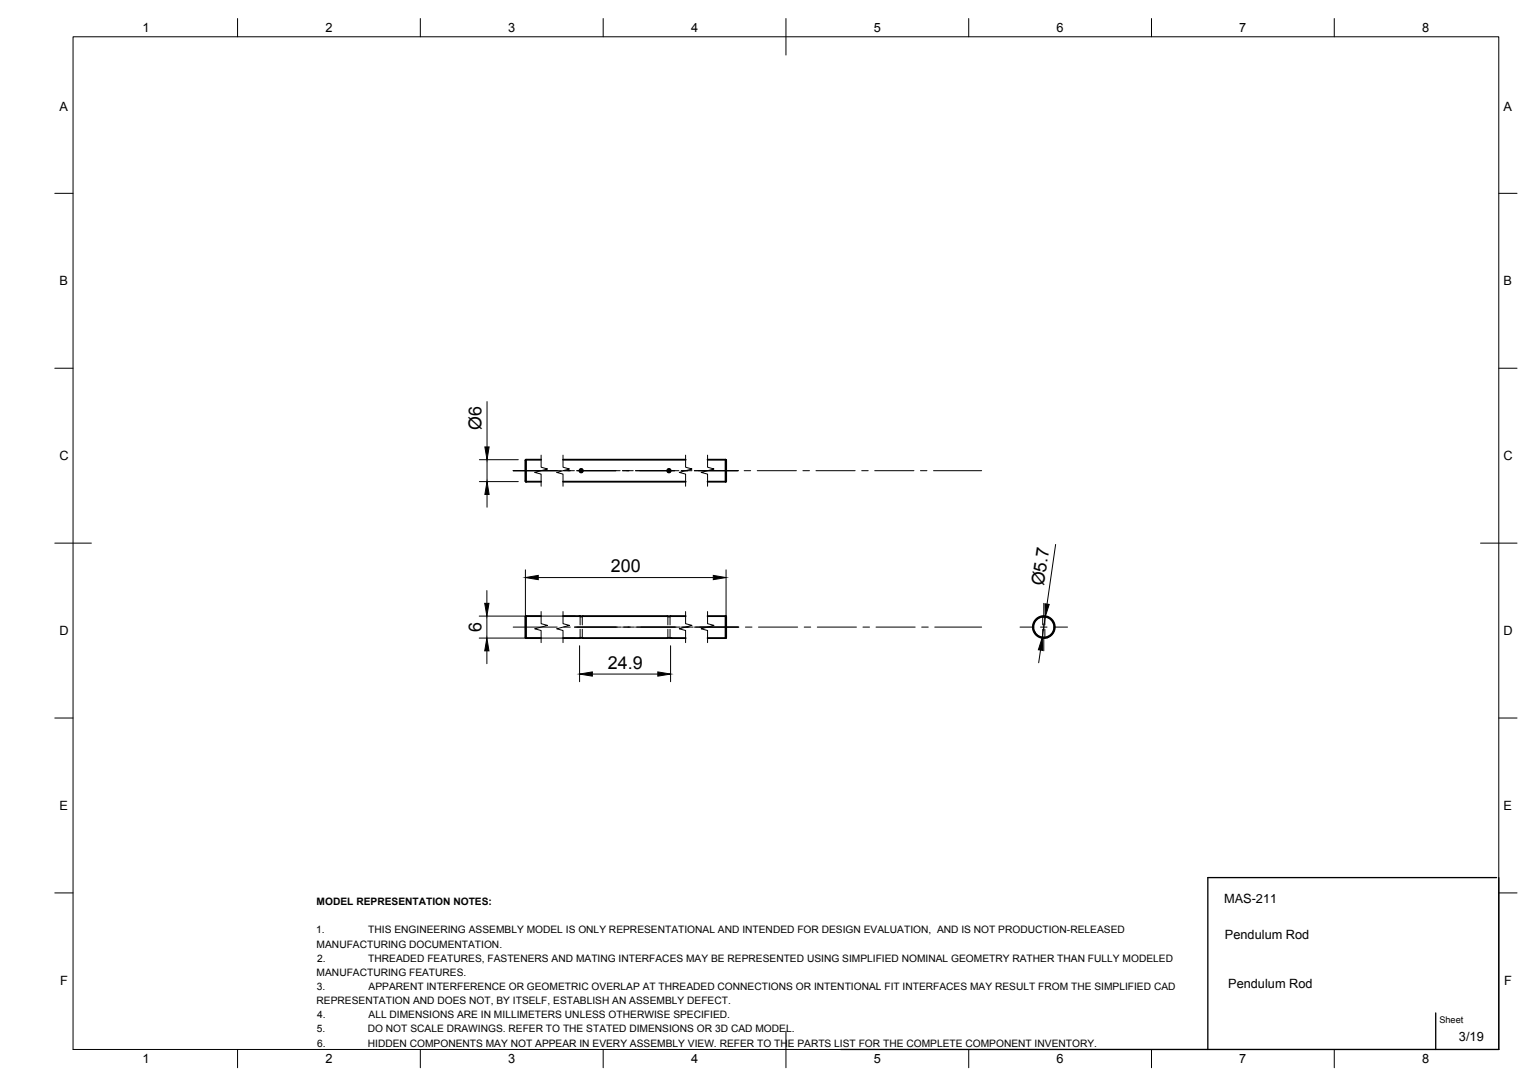
ISO-10303-21;
HEADER;
FILE_DESCRIPTION(
 (''),
 '2;1');
FILE_NAME ( 'Pendulum Rod.step', '2026-10-05T20:07:59+06:00', ( '' ), ( '' ), 'STEP AP214', 'Unspecified', '' );
FILE_SCHEMA (('AUTOMOTIVE_DESIGN { 1 0 10303 214 3 1 1 }'));
ENDSEC;
DATA;
#10=MECHANICAL_DESIGN_GEOMETRIC_PRESENTATION_REPRESENTATION('',(#319),#196741);
#319=STYLED_ITEM('',(#196765),#338) ;
#338=MANIFOLD_SOLID_BREP('Pendulum Rod',#8715) ;
#357=PLANE('',#8753) ;
#358=PLANE('',#8754) ;
#554=FACE_BOUND('',#1339,.T.) ;
#555=FACE_BOUND('',#1340,.T.) ;
#556=FACE_BOUND('',#1341,.T.) ;
#557=FACE_BOUND('',#1342,.T.) ;
#612=CIRCLE('',#8751,2.99999999999999) ;
#613=CIRCLE('',#8752,2.99999999999999) ;
#811=B_SPLINE_SURFACE_WITH_KNOTS('',1,3,((#12126,#12127,#12128,#12129,#12130,
#12131,#12132,#12133,#12134,#12135,#12136,#12137,#12138,#12139,#12140),
(#12141,#12142,#12143,#12144,#12145,#12146,#12147,#12148,#12149,#12150,
#12151,#12152,#12153,#12154,#12155)),.UNSPECIFIED.,.F.,.T.,.F.,(2,2),(4,
1,1,1,1,1,1,1,1,1,1,1,4),(-8.8354979436913E-5,0.241230871771051),(0.,0.433069184072941,
0.613631069879533,0.707969844415473,0.800502285413489,0.982878828682618,
1.41593872955056,1.84899944094778,2.03137686036412,2.12390982409441,2.21644278782049,
2.39882020722706,2.83187996119986),.UNSPECIFIED.) ;
#812=B_SPLINE_SURFACE_WITH_KNOTS('',1,3,((#12173,#12174,#12175,#12176,#12177,
#12178,#12179,#12180,#12181,#12182,#12183,#12184,#12185,#12186,#12187),
(#12188,#12189,#12190,#12191,#12192,#12193,#12194,#12195,#12196,#12197,
#12198,#12199,#12200,#12201,#12202)),.UNSPECIFIED.,.F.,.T.,.F.,(2,2),(4,
1,1,1,1,1,1,1,1,1,1,1,4),(-8.82843032138443E-5,0.241231935350036),(0.,0.433059753999551,
0.615437173415573,0.707970137120889,0.802309447772199,0.982872196325326,
1.41594123358707,1.84900113443533,2.03137767770577,2.12391011870702,2.21824889324341,
2.39881077905672,2.83187996310763),.UNSPECIFIED.) ;
#813=B_SPLINE_SURFACE_WITH_KNOTS('',1,3,((#12220,#12221,#12222,#12223,#12224,
#12225,#12226,#12227,#12228,#12229,#12230,#12231,#12232,#12233,#12234),
(#12235,#12236,#12237,#12238,#12239,#12240,#12241,#12242,#12243,#12244,
#12245,#12246,#12247,#12248,#12249)),.UNSPECIFIED.,.F.,.T.,.F.,(2,2),(4,
1,1,1,1,1,1,1,1,1,1,1,4),(-8.85365464214024E-5,0.241919354715635),(0.,0.433059753978827,
0.615437173388124,0.707970137104854,0.802309447755686,0.982872196316439,
1.41594123355621,1.84900113442618,2.03137767770062,2.12391011869139,2.21824889322736,
2.39881077903564,2.83187996310738),.UNSPECIFIED.) ;
#814=B_SPLINE_SURFACE_WITH_KNOTS('',1,3,((#12267,#12268,#12269,#12270,#12271,
#12272,#12273,#12274,#12275,#12276,#12277,#12278,#12279,#12280,#12281),
(#12282,#12283,#12284,#12285,#12286,#12287,#12288,#12289,#12290,#12291,
#12292,#12293,#12294,#12295,#12296)),.UNSPECIFIED.,.F.,.T.,.F.,(2,2),(4,
1,1,1,1,1,1,1,1,1,1,1,4),(-8.86192306118932E-5,0.241918274947197),(0.,0.433069184052406,
0.61363106986425,0.707969844400602,0.800502285411225,0.982878828678875,
1.41593872952055,1.849007766784,2.02957051533547,2.12390982598676,2.21644278969928,
2.39882020911001,2.83187996310763),.UNSPECIFIED.) ;
#815=B_SPLINE_SURFACE_WITH_KNOTS('',1,3,((#12362,#12363,#12364,#12365,#12366,
#12367,#12368,#12369,#12370,#12371,#12372,#12373,#12374,#12375,#12376,#12377,
#12378,#12379,#12380),(#12381,#12382,#12383,#12384,#12385,#12386,#12387,
#12388,#12389,#12390,#12391,#12392,#12393,#12394,#12395,#12396,#12397,#12398,
#12399)),.UNSPECIFIED.,.F.,.T.,.F.,(2,2),(4,1,1,1,1,1,1,1,1,1,1,1,1,1,1,
1,4),(0.,0.214916064382941),(0.,1.11916410687735,2.23832821375471,3.35749232063191,
4.47665642750911,5.59582053438647,6.71498464126383,7.83414874814102,8.95331285501821,
10.0724769618908,11.1916410687635,12.3108051756408,13.4299692825182,14.5491333893954,
15.6682974962725,16.7874616031499,17.9066257100273),.UNSPECIFIED.) ;
#816=B_SPLINE_SURFACE_WITH_KNOTS('',3,1,((#12401,#12402),(#12403,#12404),
(#12405,#12406),(#12407,#12408),(#12409,#12410),(#12411,#12412),(#12413,
#12414),(#12415,#12416),(#12417,#12418),(#12419,#12420),(#12421,#12422),
(#12423,#12424),(#12425,#12426),(#12427,#12428),(#12429,#12430),(#12431,
#12432),(#12433,#12434),(#12435,#12436),(#12437,#12438)),.UNSPECIFIED.,
 .T.,.F.,.F.,(4,1,1,1,1,1,1,1,1,1,1,1,1,1,1,1,4),(2,2),(0.,1.11916410687736,
2.23832821375472,3.35749232063194,4.47665642750915,5.5958205343865,6.71498464126385,
7.83414874813648,8.95331285500911,10.0724769618863,11.1916410687635,12.3108051756408,
13.4299692825181,14.5491333893953,15.6682974962725,16.7874616031499,17.9066257100273),
(0.,0.214916064382901),.UNSPECIFIED.) ;
#859=FACE_OUTER_BOUND('',#1332,.T.) ;
#860=FACE_OUTER_BOUND('',#1333,.T.) ;
#861=FACE_OUTER_BOUND('',#1334,.T.) ;
#862=FACE_OUTER_BOUND('',#1335,.T.) ;
#863=FACE_OUTER_BOUND('',#1336,.T.) ;
#864=FACE_OUTER_BOUND('',#1337,.T.) ;
#865=FACE_OUTER_BOUND('',#1338,.T.) ;
#866=FACE_OUTER_BOUND('',#1343,.T.) ;
#867=FACE_OUTER_BOUND('',#1344,.T.) ;
#868=FACE_OUTER_BOUND('',#1345,.T.) ;
#869=FACE_OUTER_BOUND('',#1346,.T.) ;
#1332=EDGE_LOOP('',(#5568,#5569,#5570,#5571,#5572,#5573)) ;
#1333=EDGE_LOOP('',(#5574,#5575,#5576,#5577,#5578,#5579)) ;
#1334=EDGE_LOOP('',(#5580,#5581,#5582,#5583,#5584)) ;
#1335=EDGE_LOOP('',(#5585,#5586,#5587,#5588,#5589)) ;
#1336=EDGE_LOOP('',(#5590,#5591,#5592,#5593,#5594)) ;
#1337=EDGE_LOOP('',(#5595,#5596,#5597,#5598,#5599)) ;
#1338=EDGE_LOOP('',(#5600,#5601,#5602,#5603)) ;
#1339=EDGE_LOOP('',(#5604)) ;
#1340=EDGE_LOOP('',(#5605)) ;
#1341=EDGE_LOOP('',(#5606)) ;
#1342=EDGE_LOOP('',(#5607)) ;
#1343=EDGE_LOOP('',(#5608)) ;
#1344=EDGE_LOOP('',(#5609)) ;
#1345=EDGE_LOOP('',(#5610,#5611,#5612,#5613)) ;
#1346=EDGE_LOOP('',(#5614,#5615,#5616,#5617)) ;
#1863=LINE('',#11652,#2566) ;
#1864=LINE('',#11926,#2567) ;
#1865=LINE('',#12157,#2568) ;
#1866=LINE('',#12204,#2569) ;
#1867=LINE('',#12251,#2570) ;
#1868=LINE('',#12298,#2571) ;
#1869=LINE('',#12318,#2572) ;
#1870=LINE('',#12400,#2573) ;
#1871=LINE('',#12439,#2574) ;
#2566=VECTOR('',#9461,0.300000000000011) ;
#2567=VECTOR('',#9464,0.299999999999991) ;
#2568=VECTOR('',#9465,10.) ;
#2569=VECTOR('',#9466,10.) ;
#2570=VECTOR('',#9467,10.) ;
#2571=VECTOR('',#9468,10.) ;
#2572=VECTOR('',#9473,3.00000000000003) ;
#2573=VECTOR('',#9480,10.) ;
#2574=VECTOR('',#9481,10.) ;
#3269=B_SPLINE_CURVE_WITH_KNOTS('',3,(#11581,#11582,#11583,#11584,#11585,
#11586,#11587,#11588,#11589,#11590,#11591,#11592,#11593,#11594,#11595,#11596,
#11597,#11598,#11599,#11600,#11601,#11602,#11603,#11604,#11605,#11606,#11607,
#11608,#11609,#11610,#11611,#11612,#11613,#11614,#11615,#11616,#11617,#11618,
#11619,#11620,#11621,#11622,#11623,#11624,#11625,#11626,#11627,#11628,#11629,
#11630,#11631,#11632,#11633,#11634,#11635,#11636,#11637,#11638,#11639,#11640,
#11641,#11642,#11643,#11644,#11645,#11646,#11647,#11648,#11649,#11650),
 .UNSPECIFIED.,.F.,.F.,(4,3,3,3,3,3,3,3,3,3,3,3,3,3,3,3,3,3,3,3,3,3,3,4),
(0.,0.0793197138435201,0.158771385884217,0.238558484111915,0.306313523372651,
0.403832448656896,0.433069184072941,0.511729267835096,0.590263878581832,
0.613631069879533,0.690390876330624,0.707969844415473,0.800502285413489,
0.876862882016797,0.95333936184816,0.982878828682618,1.06189090503122,1.14078623960736,
1.21960243454601,1.29840986633391,1.32860366242735,1.39861936931628,1.41593872955056,
1.41596897684906),.UNSPECIFIED.) ;
#3270=B_SPLINE_CURVE_WITH_KNOTS('',3,(#11654,#11655,#11656,#11657,#11658,
#11659,#11660,#11661,#11662,#11663,#11664,#11665,#11666,#11667,#11668,#11669,
#11670,#11671,#11672,#11673,#11674,#11675,#11676,#11677,#11678,#11679,#11680,
#11681,#11682,#11683,#11684,#11685,#11686,#11687,#11688,#11689,#11690,#11691,
#11692,#11693,#11694,#11695,#11696,#11697,#11698,#11699,#11700,#11701,#11702,
#11703,#11704,#11705,#11706,#11707,#11708,#11709,#11710,#11711,#11712,#11713,
#11714,#11715,#11716,#11717),.UNSPECIFIED.,.F.,.F.,(4,3,3,3,3,3,3,3,3,3,
3,3,3,3,3,3,3,3,3,3,3,4),(1.41596880340121,1.49262148871634,1.5668573581781,
1.64471845141992,1.72257954466174,1.80445466514378,1.84900113443533,1.92515260613569,
2.0012049728828,2.03137767770577,2.12391011870702,2.19942692290802,2.21824889324341,
2.29711576720828,2.37613469075668,2.39881077905672,2.48964910629467,2.58046623905025,
2.67010886019969,2.72490396964329,2.79646171749926,2.83187996310763),
 .UNSPECIFIED.) ;
#3271=B_SPLINE_CURVE_WITH_KNOTS('',3,(#11718,#11719,#11720,#11721,#11722,
#11723,#11724,#11725,#11726,#11727,#11728,#11729,#11730,#11731,#11732,#11733,
#11734,#11735,#11736,#11737,#11738,#11739,#11740,#11741,#11742,#11743,#11744,
#11745,#11746,#11747,#11748,#11749,#11750,#11751,#11752,#11753,#11754,#11755,
#11756,#11757,#11758,#11759,#11760,#11761,#11762,#11763,#11764,#11765,#11766,
#11767,#11768,#11769,#11770,#11771,#11772,#11773,#11774,#11775,#11776,#11777,
#11778,#11779,#11780,#11781,#11782,#11783,#11784,#11785,#11786,#11787),
 .UNSPECIFIED.,.F.,.F.,(4,3,3,3,3,3,3,3,3,3,3,3,3,3,3,3,3,3,3,3,3,3,3,4),
(0.,0.0793133374912053,0.158758235390486,0.238538175205765,0.306301524869595,
0.403803180865383,0.433059753999551,0.511690783685005,0.590197964800243,
0.615437173415573,0.692151852374993,0.707970137120889,0.802309447772199,
0.878720775265787,0.955248849211538,0.982872196325326,1.06188787249591,
1.14078682148802,1.21960661441308,1.2984175189742,1.32858362623266,1.39860014615873,
1.41594123358707,1.41596880340121),.UNSPECIFIED.) ;
#3272=B_SPLINE_CURVE_WITH_KNOTS('',3,(#11788,#11789,#11790,#11791,#11792,
#11793,#11794,#11795,#11796,#11797,#11798,#11799,#11800,#11801,#11802,#11803,
#11804,#11805,#11806,#11807,#11808,#11809,#11810,#11811,#11812,#11813,#11814,
#11815,#11816,#11817,#11818,#11819,#11820,#11821,#11822,#11823,#11824,#11825,
#11826,#11827,#11828,#11829,#11830,#11831,#11832,#11833,#11834,#11835,#11836,
#11837,#11838,#11839,#11840,#11841,#11842,#11843,#11844,#11845,#11846,#11847,
#11848,#11849,#11850,#11851),.UNSPECIFIED.,.F.,.F.,(4,3,3,3,3,3,3,3,3,3,
3,3,3,3,3,3,3,3,3,3,3,4),(1.41596897684906,1.49265653903016,1.56689293584109,
1.64480608070727,1.72271922557345,1.80458348138907,1.84899944094778,1.92515534328894,
2.0012121330888,2.03137686036412,2.12390982409441,2.19935680708818,2.21644278782049,
2.2952634447841,2.37423511805567,2.39882020722706,2.48964792234117,2.58045374598227,
2.6700867011423,2.72489655815223,2.79645311316558,2.83187996119986),
 .UNSPECIFIED.) ;
#3273=B_SPLINE_CURVE_WITH_KNOTS('',3,(#11855,#11856,#11857,#11858,#11859,
#11860,#11861,#11862,#11863,#11864,#11865,#11866,#11867,#11868,#11869,#11870,
#11871,#11872,#11873,#11874,#11875,#11876,#11877,#11878,#11879,#11880,#11881,
#11882,#11883,#11884,#11885,#11886,#11887,#11888,#11889,#11890,#11891,#11892,
#11893,#11894,#11895,#11896,#11897,#11898,#11899,#11900,#11901,#11902,#11903,
#11904,#11905,#11906,#11907,#11908,#11909,#11910,#11911,#11912,#11913,#11914,
#11915,#11916,#11917,#11918,#11919,#11920,#11921,#11922,#11923,#11924),
 .UNSPECIFIED.,.F.,.F.,(4,3,3,3,3,3,3,3,3,3,3,3,3,3,3,3,3,3,3,3,3,3,3,4),
(0.,0.0793133370868211,0.158758234556949,0.238538173913318,0.306301520321067,
0.403803175477182,0.433059753978827,0.511690783698259,0.590197964845532,
0.615437173388124,0.692151852363811,0.707970137104854,0.802309447755686,
0.87872077528125,0.955248849259362,0.982872196316439,1.06188787193309,1.14078682038421,
1.21960661277611,1.29841751684233,1.32858364651257,1.39860016603356,1.41594123355621,
1.41596880335427),.UNSPECIFIED.) ;
#3274=B_SPLINE_CURVE_WITH_KNOTS('',3,(#11928,#11929,#11930,#11931,#11932,
#11933,#11934,#11935,#11936,#11937,#11938,#11939,#11940,#11941,#11942,#11943,
#11944,#11945,#11946,#11947,#11948,#11949,#11950,#11951,#11952,#11953,#11954,
#11955,#11956,#11957,#11958,#11959,#11960,#11961,#11962,#11963,#11964,#11965,
#11966,#11967,#11968,#11969,#11970,#11971,#11972,#11973,#11974,#11975,#11976,
#11977,#11978,#11979,#11980,#11981,#11982,#11983,#11984,#11985,#11986,#11987,
#11988,#11989,#11990,#11991),.UNSPECIFIED.,.F.,.F.,(4,3,3,3,3,3,3,3,3,3,
3,3,3,3,3,3,3,3,3,3,3,4),(1.41596956338659,1.49266311646134,1.56690058990888,
1.64482218279723,1.72274377568557,1.80460850560754,1.849007766784,1.92524484137593,
2.00137969415775,2.02957051533547,2.12390982598676,2.19939955812894,2.21644278969928,
2.29526521978404,2.37423861455297,2.39882020911001,2.48964647817264,2.58045077014705,
2.67008242771561,2.72489376468843,2.79645019556297,2.83187996310763),
 .UNSPECIFIED.) ;
#3275=B_SPLINE_CURVE_WITH_KNOTS('',3,(#11992,#11993,#11994,#11995,#11996,
#11997,#11998,#11999,#12000,#12001,#12002,#12003,#12004,#12005,#12006,#12007,
#12008,#12009,#12010,#12011,#12012,#12013,#12014,#12015,#12016,#12017,#12018,
#12019,#12020,#12021,#12022,#12023,#12024,#12025,#12026,#12027,#12028,#12029,
#12030,#12031,#12032,#12033,#12034,#12035,#12036,#12037,#12038,#12039,#12040,
#12041,#12042,#12043,#12044,#12045,#12046,#12047,#12048,#12049,#12050,#12051,
#12052,#12053,#12054,#12055,#12056,#12057,#12058,#12059,#12060,#12061),
 .UNSPECIFIED.,.F.,.F.,(4,3,3,3,3,3,3,3,3,3,3,3,3,3,3,3,3,3,3,3,3,3,3,4),
(0.,0.0793198911693566,0.158771759312593,0.238559074159999,0.306312735619829,
0.403832566518769,0.433069184052406,0.511730463050406,0.590266238023745,
0.61363106986425,0.690383033927815,0.707969844400602,0.800502285411225,
0.876854197724648,0.953321820846053,0.982878828678875,1.06189673932164,
1.14079797822371,1.21962007756801,1.29843326555185,1.32859538269108,1.3986125617673,
1.41593872952055,1.41596956338659),.UNSPECIFIED.) ;
#3276=B_SPLINE_CURVE_WITH_KNOTS('',3,(#12062,#12063,#12064,#12065,#12066,
#12067,#12068,#12069,#12070,#12071,#12072,#12073,#12074,#12075,#12076,#12077,
#12078,#12079,#12080,#12081,#12082,#12083,#12084,#12085,#12086,#12087,#12088,
#12089,#12090,#12091,#12092,#12093,#12094,#12095,#12096,#12097,#12098,#12099,
#12100,#12101,#12102,#12103,#12104,#12105,#12106,#12107,#12108,#12109,#12110,
#12111,#12112,#12113,#12114,#12115,#12116,#12117,#12118,#12119,#12120,#12121,
#12122,#12123,#12124,#12125),.UNSPECIFIED.,.F.,.F.,(4,3,3,3,3,3,3,3,3,3,
3,3,3,3,3,3,3,3,3,3,3,4),(1.41596880335427,1.49262163677989,1.56685751827755,
1.64471882766714,1.72258013705673,1.80445525976957,1.84900113442618,1.92515260611125,
2.00120497284308,2.03137767770062,2.12391011869139,2.19942692303724,2.21824889322736,
2.29711576705383,2.37613469046074,2.39881077903564,2.48964909647063,2.58046621914314,
2.67010883124273,2.72490414691485,2.79646188868388,2.83187996310738),
 .UNSPECIFIED.) ;
#3277=B_SPLINE_CURVE_WITH_KNOTS('',3,(#12158,#12159,#12160,#12161,#12162,
#12163,#12164,#12165,#12166,#12167,#12168,#12169,#12170,#12171,#12172),
 .UNSPECIFIED.,.T.,.F.,(4,1,1,1,1,1,1,1,1,1,1,1,4),(0.,0.433069184072941,
0.613631069879533,0.707969844415473,0.800502285413489,0.982878828682618,
1.41593872955056,1.84899944094778,2.03137686036412,2.12390982409441,2.21644278782049,
2.39882020722706,2.83187996119986),.UNSPECIFIED.) ;
#3278=B_SPLINE_CURVE_WITH_KNOTS('',3,(#12205,#12206,#12207,#12208,#12209,
#12210,#12211,#12212,#12213,#12214,#12215,#12216,#12217,#12218,#12219),
 .UNSPECIFIED.,.T.,.F.,(4,1,1,1,1,1,1,1,1,1,1,1,4),(0.,0.433059753999551,
0.615437173415573,0.707970137120889,0.802309447772199,0.982872196325326,
1.41594123358707,1.84900113443533,2.03137767770577,2.12391011870702,2.21824889324341,
2.39881077905672,2.83187996310763),.UNSPECIFIED.) ;
#3279=B_SPLINE_CURVE_WITH_KNOTS('',3,(#12252,#12253,#12254,#12255,#12256,
#12257,#12258,#12259,#12260,#12261,#12262,#12263,#12264,#12265,#12266),
 .UNSPECIFIED.,.T.,.F.,(4,1,1,1,1,1,1,1,1,1,1,1,4),(0.,0.433059753978827,
0.615437173388124,0.707970137104854,0.802309447755686,0.982872196316439,
1.41594123355621,1.84900113442618,2.03137767770062,2.12391011869139,2.21824889322736,
2.39881077903564,2.83187996310738),.UNSPECIFIED.) ;
#3280=B_SPLINE_CURVE_WITH_KNOTS('',3,(#12299,#12300,#12301,#12302,#12303,
#12304,#12305,#12306,#12307,#12308,#12309,#12310,#12311,#12312,#12313),
 .UNSPECIFIED.,.T.,.F.,(4,1,1,1,1,1,1,1,1,1,1,1,4),(0.,0.433069184052406,
0.61363106986425,0.707969844400602,0.800502285411225,0.982878828678875,
1.41593872952055,1.849007766784,2.02957051533547,2.12390982598676,2.21644278969928,
2.39882020911001,2.83187996310763),.UNSPECIFIED.) ;
#3281=B_SPLINE_CURVE_WITH_KNOTS('',3,(#12322,#12323,#12324,#12325,#12326,
#12327,#12328,#12329,#12330,#12331,#12332,#12333,#12334,#12335,#12336,#12337,
#12338,#12339,#12340),.UNSPECIFIED.,.T.,.F.,(4,1,1,1,1,1,1,1,1,1,1,1,1,
1,1,1,4),(0.,1.11916410687735,2.23832821375471,3.35749232063191,4.47665642750911,
5.59582053438647,6.71498464126383,7.83414874814102,8.95331285501821,10.0724769618908,
11.1916410687635,12.3108051756408,13.4299692825182,14.5491333893954,15.6682974962725,
16.7874616031499,17.9066257100273),.UNSPECIFIED.) ;
#3282=B_SPLINE_CURVE_WITH_KNOTS('',3,(#12343,#12344,#12345,#12346,#12347,
#12348,#12349,#12350,#12351,#12352,#12353,#12354,#12355,#12356,#12357,#12358,
#12359,#12360,#12361),.UNSPECIFIED.,.T.,.F.,(4,1,1,1,1,1,1,1,1,1,1,1,1,
1,1,1,4),(0.,1.11916410687736,2.23832821375472,3.35749232063194,4.47665642750915,
5.5958205343865,6.71498464126385,7.83414874813648,8.95331285500911,10.0724769618863,
11.1916410687635,12.3108051756408,13.4299692825181,14.5491333893953,15.6682974962725,
16.7874616031499,17.9066257100273),.UNSPECIFIED.) ;
#3447=VERTEX_POINT('',#11579) ;
#3448=VERTEX_POINT('',#11580) ;
#3449=VERTEX_POINT('',#11651) ;
#3450=VERTEX_POINT('',#11653) ;
#3451=VERTEX_POINT('',#11853) ;
#3452=VERTEX_POINT('',#11854) ;
#3453=VERTEX_POINT('',#11925) ;
#3454=VERTEX_POINT('',#11927) ;
#3455=VERTEX_POINT('',#12156) ;
#3456=VERTEX_POINT('',#12203) ;
#3457=VERTEX_POINT('',#12250) ;
#3458=VERTEX_POINT('',#12297) ;
#3459=VERTEX_POINT('',#12315) ;
#3460=VERTEX_POINT('',#12317) ;
#3461=VERTEX_POINT('',#12321) ;
#3462=VERTEX_POINT('',#12342) ;
#4292=EDGE_CURVE('',#3447,#3448,#3269,.T.) ;
#4293=EDGE_CURVE('',#3448,#3449,#1863,.T.) ;
#4294=EDGE_CURVE('',#3449,#3450,#3270,.T.) ;
#4295=EDGE_CURVE('',#3450,#3449,#3271,.T.) ;
#4296=EDGE_CURVE('',#3448,#3447,#3272,.T.) ;
#4297=EDGE_CURVE('',#3451,#3452,#3273,.T.) ;
#4298=EDGE_CURVE('',#3452,#3453,#1864,.T.) ;
#4299=EDGE_CURVE('',#3453,#3454,#3274,.T.) ;
#4300=EDGE_CURVE('',#3454,#3453,#3275,.T.) ;
#4301=EDGE_CURVE('',#3452,#3451,#3276,.T.) ;
#4302=EDGE_CURVE('',#3447,#3455,#1865,.T.) ;
#4303=EDGE_CURVE('',#3455,#3455,#3277,.T.) ;
#4304=EDGE_CURVE('',#3450,#3456,#1866,.T.) ;
#4305=EDGE_CURVE('',#3456,#3456,#3278,.T.) ;
#4306=EDGE_CURVE('',#3451,#3457,#1867,.T.) ;
#4307=EDGE_CURVE('',#3457,#3457,#3279,.T.) ;
#4308=EDGE_CURVE('',#3454,#3458,#1868,.T.) ;
#4309=EDGE_CURVE('',#3458,#3458,#3280,.T.) ;
#4310=EDGE_CURVE('',#3459,#3459,#612,.T.) ;
#4311=EDGE_CURVE('',#3459,#3460,#1869,.T.) ;
#4312=EDGE_CURVE('',#3460,#3460,#613,.T.) ;
#4313=EDGE_CURVE('',#3461,#3461,#3281,.T.) ;
#4314=EDGE_CURVE('',#3462,#3462,#3282,.T.) ;
#4315=EDGE_CURVE('',#3459,#3461,#1870,.T.) ;
#4316=EDGE_CURVE('',#3460,#3462,#1871,.T.) ;
#5568=ORIENTED_EDGE('',*,*,#4292,.T.) ;
#5569=ORIENTED_EDGE('',*,*,#4293,.T.) ;
#5570=ORIENTED_EDGE('',*,*,#4294,.T.) ;
#5571=ORIENTED_EDGE('',*,*,#4295,.T.) ;
#5572=ORIENTED_EDGE('',*,*,#4293,.F.) ;
#5573=ORIENTED_EDGE('',*,*,#4296,.T.) ;
#5574=ORIENTED_EDGE('',*,*,#4297,.T.) ;
#5575=ORIENTED_EDGE('',*,*,#4298,.T.) ;
#5576=ORIENTED_EDGE('',*,*,#4299,.T.) ;
#5577=ORIENTED_EDGE('',*,*,#4300,.T.) ;
#5578=ORIENTED_EDGE('',*,*,#4298,.F.) ;
#5579=ORIENTED_EDGE('',*,*,#4301,.T.) ;
#5580=ORIENTED_EDGE('',*,*,#4302,.T.) ;
#5581=ORIENTED_EDGE('',*,*,#4303,.T.) ;
#5582=ORIENTED_EDGE('',*,*,#4302,.F.) ;
#5583=ORIENTED_EDGE('',*,*,#4296,.F.) ;
#5584=ORIENTED_EDGE('',*,*,#4292,.F.) ;
#5585=ORIENTED_EDGE('',*,*,#4304,.T.) ;
#5586=ORIENTED_EDGE('',*,*,#4305,.T.) ;
#5587=ORIENTED_EDGE('',*,*,#4304,.F.) ;
#5588=ORIENTED_EDGE('',*,*,#4294,.F.) ;
#5589=ORIENTED_EDGE('',*,*,#4295,.F.) ;
#5590=ORIENTED_EDGE('',*,*,#4306,.T.) ;
#5591=ORIENTED_EDGE('',*,*,#4307,.T.) ;
#5592=ORIENTED_EDGE('',*,*,#4306,.F.) ;
#5593=ORIENTED_EDGE('',*,*,#4301,.F.) ;
#5594=ORIENTED_EDGE('',*,*,#4297,.F.) ;
#5595=ORIENTED_EDGE('',*,*,#4308,.T.) ;
#5596=ORIENTED_EDGE('',*,*,#4309,.T.) ;
#5597=ORIENTED_EDGE('',*,*,#4308,.F.) ;
#5598=ORIENTED_EDGE('',*,*,#4299,.F.) ;
#5599=ORIENTED_EDGE('',*,*,#4300,.F.) ;
#5600=ORIENTED_EDGE('',*,*,#4310,.T.) ;
#5601=ORIENTED_EDGE('',*,*,#4311,.T.) ;
#5602=ORIENTED_EDGE('',*,*,#4312,.F.) ;
#5603=ORIENTED_EDGE('',*,*,#4311,.F.) ;
#5604=ORIENTED_EDGE('',*,*,#4307,.F.) ;
#5605=ORIENTED_EDGE('',*,*,#4305,.F.) ;
#5606=ORIENTED_EDGE('',*,*,#4303,.F.) ;
#5607=ORIENTED_EDGE('',*,*,#4309,.F.) ;
#5608=ORIENTED_EDGE('',*,*,#4313,.F.) ;
#5609=ORIENTED_EDGE('',*,*,#4314,.T.) ;
#5610=ORIENTED_EDGE('',*,*,#4315,.T.) ;
#5611=ORIENTED_EDGE('',*,*,#4313,.T.) ;
#5612=ORIENTED_EDGE('',*,*,#4315,.F.) ;
#5613=ORIENTED_EDGE('',*,*,#4310,.F.) ;
#5614=ORIENTED_EDGE('',*,*,#4312,.T.) ;
#5615=ORIENTED_EDGE('',*,*,#4316,.T.) ;
#5616=ORIENTED_EDGE('',*,*,#4314,.F.) ;
#5617=ORIENTED_EDGE('',*,*,#4316,.F.) ;
#8120=CYLINDRICAL_SURFACE('',#8748,0.300000000000011) ;
#8121=CYLINDRICAL_SURFACE('',#8749,0.299999999999991) ;
#8122=CYLINDRICAL_SURFACE('',#8750,3.00000000000003) ;
#8242=ADVANCED_FACE('',(#859),#8120,.F.) ;
#8243=ADVANCED_FACE('',(#860),#8121,.F.) ;
#8244=ADVANCED_FACE('',(#861),#811,.T.) ;
#8245=ADVANCED_FACE('',(#862),#812,.T.) ;
#8246=ADVANCED_FACE('',(#863),#813,.T.) ;
#8247=ADVANCED_FACE('',(#864),#814,.T.) ;
#8248=ADVANCED_FACE('',(#865,#554,#555,#556,#557),#8122,.T.) ;
#8249=ADVANCED_FACE('',(#866),#357,.T.) ;
#8250=ADVANCED_FACE('',(#867),#358,.T.) ;
#8251=ADVANCED_FACE('',(#868),#815,.T.) ;
#8252=ADVANCED_FACE('',(#869),#816,.T.) ;
#8715=CLOSED_SHELL('',(#8242,#8243,#8244,#8245,#8246,#8247,#8248,#8249,
#8250,#8251,#8252)) ;
#8748=AXIS2_PLACEMENT_3D('',#11578,#9459,#9460) ;
#8749=AXIS2_PLACEMENT_3D('',#11852,#9462,#9463) ;
#8750=AXIS2_PLACEMENT_3D('',#12314,#9469,#9470) ;
#8751=AXIS2_PLACEMENT_3D('',#12316,#9471,#9472) ;
#8752=AXIS2_PLACEMENT_3D('',#12319,#9474,#9475) ;
#8753=AXIS2_PLACEMENT_3D('',#12320,#9476,#9477) ;
#8754=AXIS2_PLACEMENT_3D('',#12341,#9478,#9479) ;
#9459=DIRECTION('center_axis',(-0.946101641249535,-2.18705461187032E-30,
-0.323869857234255)) ;
#9460=DIRECTION('ref_axis',(1.6950188065742E-15,1.,0.)) ;
#9461=DIRECTION('',(0.946101641249535,2.18705461187032E-30,0.323869857234254)) ;
#9462=DIRECTION('center_axis',(-0.946101641249535,-1.74964368949631E-30,
-0.323869857234254)) ;
#9463=DIRECTION('ref_axis',(-1.69501880657431E-15,-1.,0.)) ;
#9464=DIRECTION('',(0.946101641249535,1.74964368949631E-30,0.323869857234254)) ;
#9465=DIRECTION('',(-0.668996284986547,0.707106781199264,-0.229006486057089)) ;
#9466=DIRECTION('',(0.66899348741416,0.707106781186561,0.229014658477182)) ;
#9467=DIRECTION('',(-0.668996284988301,-0.707106781199269,-0.229006486051948)) ;
#9468=DIRECTION('',(0.668993487414155,-0.707106781186567,0.22901465847718)) ;
#9469=DIRECTION('center_axis',(0.,1.,0.)) ;
#9470=DIRECTION('ref_axis',(-0.21434215188659,0.,-0.976758640568194)) ;
#9471=DIRECTION('center_axis',(0.,-1.,0.)) ;
#9472=DIRECTION('ref_axis',(0.742040051540844,0.,0.670355548876312)) ;
#9473=DIRECTION('',(0.,-1.,0.)) ;
#9474=DIRECTION('center_axis',(0.,-1.,0.)) ;
#9475=DIRECTION('ref_axis',(0.742040051540844,0.,0.670355548876312)) ;
#9476=DIRECTION('center_axis',(0.,1.,0.)) ;
#9477=DIRECTION('ref_axis',(0.,0.,1.)) ;
#9478=DIRECTION('center_axis',(0.,-1.,0.)) ;
#9479=DIRECTION('ref_axis',(0.,0.,-1.)) ;
#9480=DIRECTION('',(-0.151562789093119,0.707106781186684,-0.690672658328185)) ;
#9481=DIRECTION('',(-0.15156278909311,-0.707106781186643,-0.690672658328229)) ;
#11578=CARTESIAN_POINT('Origin',(-5.63784594171726E-6,12.,130.056019952763)) ;
#11579=CARTESIAN_POINT('',(-2.69639531535793,12.3,129.132990859662)) ;
#11580=CARTESIAN_POINT('',(-2.69662395993644,11.7,129.132912589967)) ;
#11581=CARTESIAN_POINT('Ctrl Pts',(-2.69639531535755,12.3,129.132990859662)) ;
#11582=CARTESIAN_POINT('Ctrl Pts',(-2.69077162240415,12.3,129.116167020409)) ;
#11583=CARTESIAN_POINT('Ctrl Pts',(-2.68469199795713,12.2984224191665,129.099524200288)) ;
#11584=CARTESIAN_POINT('Ctrl Pts',(-2.67835058694966,12.2953054979811,129.083291730847)) ;
#11585=CARTESIAN_POINT('Ctrl Pts',(-2.67199862621724,12.29218339141,129.067032256677)) ;
#11586=CARTESIAN_POINT('Ctrl Pts',(-2.66538421612455,12.2875170237535,129.051185110066)) ;
#11587=CARTESIAN_POINT('Ctrl Pts',(-2.65869785319305,12.2813953186066,129.035967275889)) ;
#11588=CARTESIAN_POINT('Ctrl Pts',(-2.65198326201708,12.275247769067,129.020685195612)) ;
#11589=CARTESIAN_POINT('Ctrl Pts',(-2.64519630460819,12.2676328803879,129.006038323483)) ;
#11590=CARTESIAN_POINT('Ctrl Pts',(-2.63852218903446,12.2586877093307,128.992223877476)) ;
#11591=CARTESIAN_POINT('Ctrl Pts',(-2.63285454385406,12.2510914885176,128.980492678418)) ;
#11592=CARTESIAN_POINT('Ctrl Pts',(-2.62726819434588,12.2425369009626,128.969361542656)) ;
#11593=CARTESIAN_POINT('Ctrl Pts',(-2.62187074130637,12.2331313228689,128.958934247103)) ;
#11594=CARTESIAN_POINT('Ctrl Pts',(-2.61410225905873,12.2195939996322,128.943926379541)) ;
#11595=CARTESIAN_POINT('Ctrl Pts',(-2.60671352792775,12.2042653708087,128.930342789742)) ;
#11596=CARTESIAN_POINT('Ctrl Pts',(-2.5999983071543,12.1874446308271,128.918413851356)) ;
#11597=CARTESIAN_POINT('Ctrl Pts',(-2.59798504529316,12.1824016761092,128.914837486928)) ;
#11598=CARTESIAN_POINT('Ctrl Pts',(-2.59603224850718,12.177224876733,128.911409636886)) ;
#11599=CARTESIAN_POINT('Ctrl Pts',(-2.59414765019636,12.1719230232504,128.908135975523)) ;
#11600=CARTESIAN_POINT('Ctrl Pts',(-2.58907722564732,12.1576586317889,128.899328341107)) ;
#11601=CARTESIAN_POINT('Ctrl Pts',(-2.58450466969039,12.1425004895536,128.891649109489)) ;
#11602=CARTESIAN_POINT('Ctrl Pts',(-2.58058794256455,12.1266788388559,128.885199808432)) ;
#11603=CARTESIAN_POINT('Ctrl Pts',(-2.57667746312546,12.110882425739,128.878760794845)) ;
#11604=CARTESIAN_POINT('Ctrl Pts',(-2.57342083523148,12.0944252333348,128.873548122155)) ;
#11605=CARTESIAN_POINT('Ctrl Pts',(-2.5709605467127,12.0775615159586,128.869619839075)) ;
#11606=CARTESIAN_POINT('Ctrl Pts',(-2.57022851236607,12.0725438847999,128.868451017566)) ;
#11607=CARTESIAN_POINT('Ctrl Pts',(-2.56956687301894,12.0674903983032,128.867395596478)) ;
#11608=CARTESIAN_POINT('Ctrl Pts',(-2.56897911005068,12.0624080546532,128.866454310522)) ;
#11609=CARTESIAN_POINT('Ctrl Pts',(-2.56704834434127,12.045712863951,128.863362243235)) ;
#11610=CARTESIAN_POINT('Ctrl Pts',(-2.56591702181591,12.0287200061612,128.861508378651)) ;
#11611=CARTESIAN_POINT('Ctrl Pts',(-2.56555956232846,12.011690688947,128.860928790889)) ;
#11612=CARTESIAN_POINT('Ctrl Pts',(-2.56547769957746,12.0077907595744,128.860796057949)) ;
#11613=CARTESIAN_POINT('Ctrl Pts',(-2.56543635359737,12.0038889319103,128.860729952645)) ;
#11614=CARTESIAN_POINT('Ctrl Pts',(-2.56543509258672,11.9999883515565,128.860730544395)) ;
#11615=CARTESIAN_POINT('Ctrl Pts',(-2.56542845485952,11.9794564170477,128.860733659257)) ;
#11616=CARTESIAN_POINT('Ctrl Pts',(-2.56653357884379,11.9589330509582,128.862588005132)) ;
#11617=CARTESIAN_POINT('Ctrl Pts',(-2.56882120220927,11.9387964657361,128.866240323405)) ;
#11618=CARTESIAN_POINT('Ctrl Pts',(-2.57070901888315,11.9221791405632,128.869254328)) ;
#11619=CARTESIAN_POINT('Ctrl Pts',(-2.57340054229553,11.9058576648792,128.873488140823)) ;
#11620=CARTESIAN_POINT('Ctrl Pts',(-2.57675906187904,11.8900798109946,128.878905495549)) ;
#11621=CARTESIAN_POINT('Ctrl Pts',(-2.58012267828092,11.8742780129722,128.884331071539)) ;
#11622=CARTESIAN_POINT('Ctrl Pts',(-2.58415521179501,11.8590221908532,128.890943477565)) ;
#11623=CARTESIAN_POINT('Ctrl Pts',(-2.58870394705331,11.8445394749185,128.898661349037)) ;
#11624=CARTESIAN_POINT('Ctrl Pts',(-2.59046092141454,11.8389454451205,128.901642419935)) ;
#11625=CARTESIAN_POINT('Ctrl Pts',(-2.59229475598414,11.8334664720546,128.904787970042)) ;
#11626=CARTESIAN_POINT('Ctrl Pts',(-2.59419609809682,11.8281144498417,128.908091697553)) ;
#11627=CARTESIAN_POINT('Ctrl Pts',(-2.59928180221649,11.8137988770498,128.916928497888)) ;
#11628=CARTESIAN_POINT('Ctrl Pts',(-2.60486398800593,11.8003383447438,128.926936410632)) ;
#11629=CARTESIAN_POINT('Ctrl Pts',(-2.61079581228568,11.7879509898805,128.937988632388)) ;
#11630=CARTESIAN_POINT('Ctrl Pts',(-2.61671887218773,11.7755819375581,128.949024524286)) ;
#11631=CARTESIAN_POINT('Ctrl Pts',(-2.62299039132912,11.7642834255358,128.961101212608)) ;
#11632=CARTESIAN_POINT('Ctrl Pts',(-2.62945152491257,11.7542383902569,128.974055496983)) ;
#11633=CARTESIAN_POINT('Ctrl Pts',(-2.63590617735524,11.7442034311181,128.98699678696)) ;
#11634=CARTESIAN_POINT('Ctrl Pts',(-2.64254988476032,11.7354198617474,129.000813389561)) ;
#11635=CARTESIAN_POINT('Ctrl Pts',(-2.64921409275335,11.728028674419,129.015312836051)) ;
#11636=CARTESIAN_POINT('Ctrl Pts',(-2.65587755978878,11.7206383088771,129.029810670425)) ;
#11637=CARTESIAN_POINT('Ctrl Pts',(-2.66256131921654,11.714640322129,129.044990601979)) ;
#11638=CARTESIAN_POINT('Ctrl Pts',(-2.66908955986842,11.7101287337753,129.060638863111)) ;
#11639=CARTESIAN_POINT('Ctrl Pts',(-2.67159074995444,11.7084001914828,129.066634241911)) ;
#11640=CARTESIAN_POINT('Ctrl Pts',(-2.67406905115582,11.7068893270032,129.072698192146)) ;
#11641=CARTESIAN_POINT('Ctrl Pts',(-2.67651439134326,11.7055994810325,129.078818152777)) ;
#11642=CARTESIAN_POINT('Ctrl Pts',(-2.68218483507541,11.7026084865535,129.093009590261)) ;
#11643=CARTESIAN_POINT('Ctrl Pts',(-2.68767315026768,11.7008127780343,129.107487919033)) ;
#11644=CARTESIAN_POINT('Ctrl Pts',(-2.69284221889314,11.7002201050426,129.122062838334)) ;
#11645=CARTESIAN_POINT('Ctrl Pts',(-2.69412086000923,11.7000734991237,129.125668147614)) ;
#11646=CARTESIAN_POINT('Ctrl Pts',(-2.69537996760857,11.7000002555525,129.129279369597)) ;
#11647=CARTESIAN_POINT('Ctrl Pts',(-2.69661747639193,11.7000000006677,129.13289365344)) ;
#11648=CARTESIAN_POINT('Ctrl Pts',(-2.69661963763213,11.7000000002226,129.132899965585)) ;
#11649=CARTESIAN_POINT('Ctrl Pts',(-2.69662179881363,11.7,129.132906277761)) ;
#11650=CARTESIAN_POINT('Ctrl Pts',(-2.69662395993644,11.7,129.132912589967)) ;
#11651=CARTESIAN_POINT('',(2.69661214327121,11.7,130.979127130373)) ;
#11652=CARTESIAN_POINT('',(-5.63784594223766E-6,11.7,130.056019952763)) ;
#11653=CARTESIAN_POINT('',(2.69638403966492,12.3,130.979049045863)) ;
#11654=CARTESIAN_POINT('Ctrl Pts',(2.69661214327121,11.7,130.979127130373)) ;
#11655=CARTESIAN_POINT('Ctrl Pts',(2.7020891025457,11.7,130.963130731944)) ;
#11656=CARTESIAN_POINT('Ctrl Pts',(2.70718927973337,11.7014342946098,130.946939435389)) ;
#11657=CARTESIAN_POINT('Ctrl Pts',(2.7119095593469,11.7043050991552,130.930837632166)) ;
#11658=CARTESIAN_POINT('Ctrl Pts',(2.71648101121153,11.7070853888554,130.9152435097)) ;
#11659=CARTESIAN_POINT('Ctrl Pts',(2.72069587103395,11.71121272146,130.899734122869)) ;
#11660=CARTESIAN_POINT('Ctrl Pts',(2.72455232691621,11.7166364757703,130.884564828158)) ;
#11661=CARTESIAN_POINT('Ctrl Pts',(2.72859710841077,11.7223250929191,130.868654758289)) ;
#11662=CARTESIAN_POINT('Ctrl Pts',(2.7322472787346,11.7294400178026,130.853119824288)) ;
#11663=CARTESIAN_POINT('Ctrl Pts',(2.73550668072301,11.7378640130638,130.838237316637)) ;
#11664=CARTESIAN_POINT('Ctrl Pts',(2.73876608271141,11.7462880083249,130.823354808985)) ;
#11665=CARTESIAN_POINT('Ctrl Pts',(2.74163442922915,11.7560205212514,130.809125566473)) ;
#11666=CARTESIAN_POINT('Ctrl Pts',(2.7441261790723,11.7668904353912,130.795795867812)) ;
#11667=CARTESIAN_POINT('Ctrl Pts',(2.74674638783286,11.7783207337953,130.781778973899)) ;
#11668=CARTESIAN_POINT('Ctrl Pts',(2.74895573258088,11.7910207154901,130.768740512001)) ;
#11669=CARTESIAN_POINT('Ctrl Pts',(2.75079104972321,11.8047759870922,130.756908352675)) ;
#11670=CARTESIAN_POINT('Ctrl Pts',(2.75178960579543,11.8122599306932,130.750470732566)) ;
#11671=CARTESIAN_POINT('Ctrl Pts',(2.75267765917822,11.8200556433546,130.744389568471)) ;
#11672=CARTESIAN_POINT('Ctrl Pts',(2.75346280589737,11.828124644252,130.73869670229)) ;
#11673=CARTESIAN_POINT('Ctrl Pts',(2.75480500156664,11.8419184713109,130.728964839254)) ;
#11674=CARTESIAN_POINT('Ctrl Pts',(2.75585627744475,11.8565598978607,130.720339061431)) ;
#11675=CARTESIAN_POINT('Ctrl Pts',(2.75668210855654,11.871835167371,130.712992921434)) ;
#11676=CARTESIAN_POINT('Ctrl Pts',(2.75750686491625,11.8870905573592,130.70565634184)) ;
#11677=CARTESIAN_POINT('Ctrl Pts',(2.75810663489716,11.9029774700657,130.699596445547)) ;
#11678=CARTESIAN_POINT('Ctrl Pts',(2.75856124093594,11.9192571844188,130.694943450429)) ;
#11679=CARTESIAN_POINT('Ctrl Pts',(2.7587415994758,11.9257159316846,130.693097440184)) ;
#11680=CARTESIAN_POINT('Ctrl Pts',(2.75889928098971,11.932236276286,130.691472373768)) ;
#11681=CARTESIAN_POINT('Ctrl Pts',(2.75903996599774,11.9388025611289,130.69007434979)) ;
#11682=CARTESIAN_POINT('Ctrl Pts',(2.75947141313785,11.9589397801284,130.685786945926)) ;
#11683=CARTESIAN_POINT('Ctrl Pts',(2.75973882505761,11.9794562190332,130.683647098857)) ;
#11684=CARTESIAN_POINT('Ctrl Pts',(2.75974727407528,11.9999849854668,130.683648905163)) ;
#11685=CARTESIAN_POINT('Ctrl Pts',(2.75975416941714,12.0167387511568,130.683650379311)) ;
#11686=CARTESIAN_POINT('Ctrl Pts',(2.75958781337012,12.0335208417918,130.685080532272)) ;
#11687=CARTESIAN_POINT('Ctrl Pts',(2.75928684742077,12.0500768654106,130.687940087924)) ;
#11688=CARTESIAN_POINT('Ctrl Pts',(2.75921183402169,12.054203324266,130.688652809711)) ;
#11689=CARTESIAN_POINT('Ctrl Pts',(2.75912854044863,12.0583157490574,130.689454088763)) ;
#11690=CARTESIAN_POINT('Ctrl Pts',(2.75903772786621,12.0624102439617,130.690343460518)) ;
#11691=CARTESIAN_POINT('Ctrl Pts',(2.75865720954827,12.0795667906892,130.694070061338)) ;
#11692=CARTESIAN_POINT('Ctrl Pts',(2.75814458404643,12.0963905502863,130.69934360946)) ;
#11693=CARTESIAN_POINT('Ctrl Pts',(2.75741685280201,12.11261990984,130.70604220651)) ;
#11694=CARTESIAN_POINT('Ctrl Pts',(2.75668771854481,12.1288805584159,130.712753717967)) ;
#11695=CARTESIAN_POINT('Ctrl Pts',(2.75574274873753,12.1445438866639,130.720895485112)) ;
#11696=CARTESIAN_POINT('Ctrl Pts',(2.75451370053682,12.159369543475,130.730300393157)) ;
#11697=CARTESIAN_POINT('Ctrl Pts',(2.75416100014212,12.1636240674278,130.732999322929)) ;
#11698=CARTESIAN_POINT('Ctrl Pts',(2.753784995479,12.1678097828153,130.735802011507)) ;
#11699=CARTESIAN_POINT('Ctrl Pts',(2.75338428427923,12.1719214624448,130.738703894657)) ;
#11700=CARTESIAN_POINT('Ctrl Pts',(2.75177907201284,12.1883924734382,130.750328572059)) ;
#11701=CARTESIAN_POINT('Ctrl Pts',(2.7497776751587,12.2036674747774,130.763544211412)) ;
#11702=CARTESIAN_POINT('Ctrl Pts',(2.74730616641282,12.2174775160371,130.778059876953)) ;
#11703=CARTESIAN_POINT('Ctrl Pts',(2.74483523432164,12.2312843351252,130.792572155686)) ;
#11704=CARTESIAN_POINT('Ctrl Pts',(2.74189444507797,12.2436268239637,130.808383750645)) ;
#11705=CARTESIAN_POINT('Ctrl Pts',(2.73842112100024,12.2542750535698,130.825171217944)) ;
#11706=CARTESIAN_POINT('Ctrl Pts',(2.73499271641421,12.2647855727144,130.841741577803)) ;
#11707=CARTESIAN_POINT('Ctrl Pts',(2.73104549225507,12.273645282714,130.859262643965)) ;
#11708=CARTESIAN_POINT('Ctrl Pts',(2.72652958071105,12.2806718149886,130.87739295159)) ;
#11709=CARTESIAN_POINT('Ctrl Pts',(2.72376917651805,12.284966865714,130.888475315958)) ;
#11710=CARTESIAN_POINT('Ctrl Pts',(2.72079648829852,12.2885777183418,130.899784731069)) ;
#11711=CARTESIAN_POINT('Ctrl Pts',(2.71760202350623,12.2914703716165,130.911237667668)) ;
#11712=CARTESIAN_POINT('Ctrl Pts',(2.71343032445383,12.2952479305221,130.926194227802)) ;
#11713=CARTESIAN_POINT('Ctrl Pts',(2.70888518495084,12.2977936154712,130.941381586919)) ;
#11714=CARTESIAN_POINT('Ctrl Pts',(2.70396510786262,12.2990595555217,130.956556330231)) ;
#11715=CARTESIAN_POINT('Ctrl Pts',(2.70152986494422,12.2996861456112,130.964067226)) ;
#11716=CARTESIAN_POINT('Ctrl Pts',(2.69900283215451,12.3,130.971574842711)) ;
#11717=CARTESIAN_POINT('Ctrl Pts',(2.69638403966492,12.3,130.979049045863)) ;
#11718=CARTESIAN_POINT('Ctrl Pts',(2.69638403966492,12.3,130.979049045863)) ;
#11719=CARTESIAN_POINT('Ctrl Pts',(2.69076103324602,12.3,130.995871488196)) ;
#11720=CARTESIAN_POINT('Ctrl Pts',(2.68468187264347,12.2984226929191,131.012512912544)) ;
#11721=CARTESIAN_POINT('Ctrl Pts',(2.67834076653583,12.2953062802814,131.028744053711)) ;
#11722=CARTESIAN_POINT('Ctrl Pts',(2.67198914216565,12.2921846983174,131.045002118163)) ;
#11723=CARTESIAN_POINT('Ctrl Pts',(2.6653749116115,12.2875191057773,131.060847926535)) ;
#11724=CARTESIAN_POINT('Ctrl Pts',(2.65868863600529,12.2813983887177,131.076064554073)) ;
#11725=CARTESIAN_POINT('Ctrl Pts',(2.65197416245748,12.2752518588391,131.091345354493)) ;
#11726=CARTESIAN_POINT('Ctrl Pts',(2.64518723041611,12.2676382176756,131.105991084888)) ;
#11727=CARTESIAN_POINT('Ctrl Pts',(2.6385131129551,12.2586944855711,131.119804584815)) ;
#11728=CARTESIAN_POINT('Ctrl Pts',(2.63284426241128,12.2510978735995,131.131537471902)) ;
#11729=CARTESIAN_POINT('Ctrl Pts',(2.62725672268844,12.2425426252491,131.142670181118)) ;
#11730=CARTESIAN_POINT('Ctrl Pts',(2.62185820287899,12.2331361662797,131.153098904998)) ;
#11731=CARTESIAN_POINT('Ctrl Pts',(2.6140905139445,12.2196016327727,131.168104329808)) ;
#11732=CARTESIAN_POINT('Ctrl Pts',(2.60670260441095,12.2042764153757,131.181686029092)) ;
#11733=CARTESIAN_POINT('Ctrl Pts',(2.59998827003384,12.1874596072397,131.193613809643)) ;
#11734=CARTESIAN_POINT('Ctrl Pts',(2.59797355128117,12.1824135167698,131.197192887152)) ;
#11735=CARTESIAN_POINT('Ctrl Pts',(2.59601940693364,12.1772333991662,131.200623262055)) ;
#11736=CARTESIAN_POINT('Ctrl Pts',(2.59413359107694,12.171928064592,131.203899250854)) ;
#11737=CARTESIAN_POINT('Ctrl Pts',(2.58906520381469,12.1576692544956,131.212703917461)) ;
#11738=CARTESIAN_POINT('Ctrl Pts',(2.58449456346057,12.1425172907174,131.220381171779)) ;
#11739=CARTESIAN_POINT('Ctrl Pts',(2.58057886543894,12.1267022432644,131.226829324827)) ;
#11740=CARTESIAN_POINT('Ctrl Pts',(2.57666933487568,12.1109121054562,131.233267321649)) ;
#11741=CARTESIAN_POINT('Ctrl Pts',(2.5734127985507,12.0944615861081,131.238479754618)) ;
#11742=CARTESIAN_POINT('Ctrl Pts',(2.57095099057126,12.077604774293,131.242408414304)) ;
#11743=CARTESIAN_POINT('Ctrl Pts',(2.57015954596351,12.072185491828,131.243671435852)) ;
#11744=CARTESIAN_POINT('Ctrl Pts',(2.56945012023564,12.0667243718766,131.244802124643)) ;
#11745=CARTESIAN_POINT('Ctrl Pts',(2.56882707329253,12.0612302416503,131.245799567725)) ;
#11746=CARTESIAN_POINT('Ctrl Pts',(2.56693331953243,12.0445308101071,131.248831300097)) ;
#11747=CARTESIAN_POINT('Ctrl Pts',(2.56583978787764,12.0275399677871,131.250625591239)) ;
#11748=CARTESIAN_POINT('Ctrl Pts',(2.56551894829632,12.0105187380547,131.251146954998)) ;
#11749=CARTESIAN_POINT('Ctrl Pts',(2.56545279235428,12.0070090230656,131.251254458289)) ;
#11750=CARTESIAN_POINT('Ctrl Pts',(2.5654194316577,12.003498026412,131.251308007848)) ;
#11751=CARTESIAN_POINT('Ctrl Pts',(2.56541853562656,11.9999880414362,131.251307553233)) ;
#11752=CARTESIAN_POINT('Ctrl Pts',(2.56541319175008,11.9790546995262,131.251304841935)) ;
#11753=CARTESIAN_POINT('Ctrl Pts',(2.56656382462477,11.9581302988702,131.249377613881)) ;
#11754=CARTESIAN_POINT('Ctrl Pts',(2.56894086365112,11.9376174897209,131.245582103419)) ;
#11755=CARTESIAN_POINT('Ctrl Pts',(2.57086617671789,11.9210028784109,131.242507881327)) ;
#11756=CARTESIAN_POINT('Ctrl Pts',(2.57359436233372,11.9046908810092,131.238212953675)) ;
#11757=CARTESIAN_POINT('Ctrl Pts',(2.57698748511119,11.888929144442,131.232734634183)) ;
#11758=CARTESIAN_POINT('Ctrl Pts',(2.58038579213371,11.8731433260157,131.227247944539)) ;
#11759=CARTESIAN_POINT('Ctrl Pts',(2.58445096343336,11.8579101506032,131.220574554715)) ;
#11760=CARTESIAN_POINT('Ctrl Pts',(2.58902909197395,11.8434563529271,131.212796756995)) ;
#11761=CARTESIAN_POINT('Ctrl Pts',(2.59068159970462,11.8382391528888,131.209989306145)) ;
#11762=CARTESIAN_POINT('Ctrl Pts',(2.59240080428413,11.8331232393153,131.207038360296)) ;
#11763=CARTESIAN_POINT('Ctrl Pts',(2.59417902645037,11.8281183129569,131.203949078297)) ;
#11764=CARTESIAN_POINT('Ctrl Pts',(2.59926557248941,11.8138018856694,131.195112288715)) ;
#11765=CARTESIAN_POINT('Ctrl Pts',(2.60484849396956,11.8003405866959,131.185104224137)) ;
#11766=CARTESIAN_POINT('Ctrl Pts',(2.61078097101818,11.7879525676142,131.174051718868)) ;
#11767=CARTESIAN_POINT('Ctrl Pts',(2.61670468421967,11.775582848933,131.163015541089)) ;
#11768=CARTESIAN_POINT('Ctrl Pts',(2.62297677417685,11.7642837731286,131.150938435019)) ;
#11769=CARTESIAN_POINT('Ctrl Pts',(2.62943841959953,11.7542382898846,131.137983630684)) ;
#11770=CARTESIAN_POINT('Ctrl Pts',(2.6358935823194,11.7442028848604,131.12504182337)) ;
#11771=CARTESIAN_POINT('Ctrl Pts',(2.64253774111245,11.7354189847105,131.111224601619)) ;
#11772=CARTESIAN_POINT('Ctrl Pts',(2.64920236517453,11.728027594741,131.096724463487)) ;
#11773=CARTESIAN_POINT('Ctrl Pts',(2.65586623767915,11.7206370382851,131.08222596051)) ;
#11774=CARTESIAN_POINT('Ctrl Pts',(2.66255036723862,11.7146389842908,131.067045289927)) ;
#11775=CARTESIAN_POINT('Ctrl Pts',(2.66907896661331,11.7101274655826,131.051396249006)) ;
#11776=CARTESIAN_POINT('Ctrl Pts',(2.67157789020874,11.7084006111834,131.045406333657)) ;
#11777=CARTESIAN_POINT('Ctrl Pts',(2.67405396720279,11.7068910362849,131.039347972696)) ;
#11778=CARTESIAN_POINT('Ctrl Pts',(2.67649715581827,11.7056020732647,131.033233692652)) ;
#11779=CARTESIAN_POINT('Ctrl Pts',(2.68216787636944,11.7026103480075,131.019042249027)) ;
#11780=CARTESIAN_POINT('Ctrl Pts',(2.68765653077774,11.7008139298584,131.004563843729)) ;
#11781=CARTESIAN_POINT('Ctrl Pts',(2.69282602724084,11.7002205914637,130.989988791192)) ;
#11782=CARTESIAN_POINT('Ctrl Pts',(2.69410636351323,11.7000736385305,130.986378967959)) ;
#11783=CARTESIAN_POINT('Ctrl Pts',(2.69536712310768,11.7000002331711,130.982763213871)) ;
#11784=CARTESIAN_POINT('Ctrl Pts',(2.69660623340049,11.7000000005547,130.97914439066)) ;
#11785=CARTESIAN_POINT('Ctrl Pts',(2.69660820340615,11.7000000001849,130.979138637256)) ;
#11786=CARTESIAN_POINT('Ctrl Pts',(2.69661017336306,11.7,130.979132883827)) ;
#11787=CARTESIAN_POINT('Ctrl Pts',(2.69661214327121,11.7,130.979127130373)) ;
#11788=CARTESIAN_POINT('Ctrl Pts',(-2.69662395993644,11.7,129.132912589967)) ;
#11789=CARTESIAN_POINT('Ctrl Pts',(-2.70210316791571,11.7,129.148916257214)) ;
#11790=CARTESIAN_POINT('Ctrl Pts',(-2.70720519533175,11.7014355895077,129.16511505006)) ;
#11791=CARTESIAN_POINT('Ctrl Pts',(-2.71192694782818,11.7043089893165,129.18122418407)) ;
#11792=CARTESIAN_POINT('Ctrl Pts',(-2.71649777889907,11.7070905466165,129.196818421657)) ;
#11793=CARTESIAN_POINT('Ctrl Pts',(-2.72071198318379,11.7112191551628,129.212327843349)) ;
#11794=CARTESIAN_POINT('Ctrl Pts',(-2.72456777165,11.7166441842152,129.227497082678)) ;
#11795=CARTESIAN_POINT('Ctrl Pts',(-2.7286145279346,11.7223379017531,129.243417617512)) ;
#11796=CARTESIAN_POINT('Ctrl Pts',(-2.73226613681452,11.7294598193962,129.258962417819)) ;
#11797=CARTESIAN_POINT('Ctrl Pts',(-2.73552647831201,11.7378924370324,129.273853640129)) ;
#11798=CARTESIAN_POINT('Ctrl Pts',(-2.73878681980949,11.7463250546687,129.288744862438)) ;
#11799=CARTESIAN_POINT('Ctrl Pts',(-2.74165560587231,11.7560678176211,129.302981665281)) ;
#11800=CARTESIAN_POINT('Ctrl Pts',(-2.74414736354406,11.7669492094914,129.316317307692)) ;
#11801=CARTESIAN_POINT('Ctrl Pts',(-2.74676548257675,11.7783824156497,129.3303292237)) ;
#11802=CARTESIAN_POINT('Ctrl Pts',(-2.74897292156973,11.7910846326551,129.343362497685)) ;
#11803=CARTESIAN_POINT('Ctrl Pts',(-2.75080654868513,11.804841448991,129.355189389573)) ;
#11804=CARTESIAN_POINT('Ctrl Pts',(-2.75180139444525,11.8123052949875,129.361606143095)) ;
#11805=CARTESIAN_POINT('Ctrl Pts',(-2.75268641904973,11.8200789640212,129.367668410619)) ;
#11806=CARTESIAN_POINT('Ctrl Pts',(-2.7534691588745,11.8281243002186,129.373344634198)) ;
#11807=CARTESIAN_POINT('Ctrl Pts',(-2.75481124983114,11.8419188876561,129.38307712524)) ;
#11808=CARTESIAN_POINT('Ctrl Pts',(-2.75586245147619,11.8565611448242,129.391703367661)) ;
#11809=CARTESIAN_POINT('Ctrl Pts',(-2.75668826024365,11.8718372879133,129.399049797183)) ;
#11810=CARTESIAN_POINT('Ctrl Pts',(-2.75751299426833,11.8870935499778,129.406386665748)) ;
#11811=CARTESIAN_POINT('Ctrl Pts',(-2.75811279370541,11.9029813776506,129.412446676533)) ;
#11812=CARTESIAN_POINT('Ctrl Pts',(-2.75856750267306,11.9192620246435,129.417099601109)) ;
#11813=CARTESIAN_POINT('Ctrl Pts',(-2.75874784386331,11.9257190586269,129.418944987974)) ;
#11814=CARTESIAN_POINT('Ctrl Pts',(-2.75890553423442,11.9322376529964,129.420569544473)) ;
#11815=CARTESIAN_POINT('Ctrl Pts',(-2.75904625010287,11.9388021643198,129.421967177062)) ;
#11816=CARTESIAN_POINT('Ctrl Pts',(-2.75947790845114,11.9589393822915,129.426254538405)) ;
#11817=CARTESIAN_POINT('Ctrl Pts',(-2.75974565709021,11.9794557280933,129.428394318667)) ;
#11818=CARTESIAN_POINT('Ctrl Pts',(-2.75975338546674,11.9999848592252,129.428392768201)) ;
#11819=CARTESIAN_POINT('Ctrl Pts',(-2.75975968681783,12.0167233375462,129.428391504025)) ;
#11820=CARTESIAN_POINT('Ctrl Pts',(-2.75959234533244,12.0334902652325,129.426964401046)) ;
#11821=CARTESIAN_POINT('Ctrl Pts',(-2.75929232930461,12.0500316612174,129.424109886153)) ;
#11822=CARTESIAN_POINT('Ctrl Pts',(-2.75922438665313,12.0537776820901,129.423463442988)) ;
#11823=CARTESIAN_POINT('Ctrl Pts',(-2.75914970817866,12.0575121447524,129.422743994089)) ;
#11824=CARTESIAN_POINT('Ctrl Pts',(-2.75906888965378,12.061232130531,129.421951871596)) ;
#11825=CARTESIAN_POINT('Ctrl Pts',(-2.75869605947647,12.078393084155,129.418297670164)) ;
#11826=CARTESIAN_POINT('Ctrl Pts',(-2.75819241407854,12.0952281482433,129.413096445186)) ;
#11827=CARTESIAN_POINT('Ctrl Pts',(-2.75747522563908,12.1114755686859,129.406468571523)) ;
#11828=CARTESIAN_POINT('Ctrl Pts',(-2.75675666310361,12.127754118347,129.399827999197)) ;
#11829=CARTESIAN_POINT('Ctrl Pts',(-2.75582383790127,12.1434421409862,129.391755596649)) ;
#11830=CARTESIAN_POINT('Ctrl Pts',(-2.75460882273409,12.1582989041564,129.382417059579)) ;
#11831=CARTESIAN_POINT('Ctrl Pts',(-2.75423056993796,12.1629240416545,129.379509830226)) ;
#11832=CARTESIAN_POINT('Ctrl Pts',(-2.75382507299212,12.1674688166651,129.376480197129)) ;
#11833=CARTESIAN_POINT('Ctrl Pts',(-2.75339055690962,12.1719265521261,129.373333961513)) ;
#11834=CARTESIAN_POINT('Ctrl Pts',(-2.75178527076731,12.1883953118562,129.361710436775)) ;
#11835=CARTESIAN_POINT('Ctrl Pts',(-2.749784179485,12.2036683820203,129.348496221254)) ;
#11836=CARTESIAN_POINT('Ctrl Pts',(-2.74731325680201,12.2174768642847,129.333982186267)) ;
#11837=CARTESIAN_POINT('Ctrl Pts',(-2.74484292966562,12.2312820184018,129.319471649481)) ;
#11838=CARTESIAN_POINT('Ctrl Pts',(-2.74190303311995,12.2436232361933,129.303662023544)) ;
#11839=CARTESIAN_POINT('Ctrl Pts',(-2.73843079462914,12.254270639284,129.286876688016)) ;
#11840=CARTESIAN_POINT('Ctrl Pts',(-2.73500340435313,12.2647805181169,129.270308155665)) ;
#11841=CARTESIAN_POINT('Ctrl Pts',(-2.73105736529469,12.2736399653289,129.252789044357)) ;
#11842=CARTESIAN_POINT('Ctrl Pts',(-2.72654271562355,12.280666652311,129.234660773318)) ;
#11843=CARTESIAN_POINT('Ctrl Pts',(-2.72378204235909,12.2849634169113,129.223575476156)) ;
#11844=CARTESIAN_POINT('Ctrl Pts',(-2.72080895358385,12.2885756232418,129.212262987302)) ;
#11845=CARTESIAN_POINT('Ctrl Pts',(-2.71761392427958,12.2914692428885,129.200806919405)) ;
#11846=CARTESIAN_POINT('Ctrl Pts',(-2.71344268022509,12.2952469840602,129.185850544814)) ;
#11847=CARTESIAN_POINT('Ctrl Pts',(-2.70889793126579,12.2977928925214,129.170663409752)) ;
#11848=CARTESIAN_POINT('Ctrl Pts',(-2.70397812212487,12.2990591076826,129.155488943472)) ;
#11849=CARTESIAN_POINT('Ctrl Pts',(-2.70154237978428,12.299685996611,129.147976235365)) ;
#11850=CARTESIAN_POINT('Ctrl Pts',(-2.69901476984933,12.3,129.140466820952)) ;
#11851=CARTESIAN_POINT('Ctrl Pts',(-2.69639531535756,12.3,129.132990859662)) ;
#11852=CARTESIAN_POINT('Origin',(-5.63784594070025E-6,-12.,130.056019952763)) ;
#11853=CARTESIAN_POINT('',(-2.69639531535792,-12.3,129.132990859662)) ;
#11854=CARTESIAN_POINT('',(-2.69662341896302,-11.7,129.132912775153)) ;
#11855=CARTESIAN_POINT('Ctrl Pts',(-2.69639531535756,-12.3,129.132990859662)) ;
#11856=CARTESIAN_POINT('Ctrl Pts',(-2.70226117920183,-12.3,129.149730166849)) ;
#11857=CARTESIAN_POINT('Ctrl Pts',(-2.70765564961494,-12.2984226929367,
129.16660597449)) ;
#11858=CARTESIAN_POINT('Ctrl Pts',(-2.71259169348251,-12.2953062803316,
129.183318096982)) ;
#11859=CARTESIAN_POINT('Ctrl Pts',(-2.7175359249746,-12.2921846984012,129.200057940576)) ;
#11860=CARTESIAN_POINT('Ctrl Pts',(-2.72201999879468,-12.2875191059108,
129.216632944885)) ;
#11861=CARTESIAN_POINT('Ctrl Pts',(-2.72606156203862,-12.2813983889147,
129.23275491124)) ;
#11862=CARTESIAN_POINT('Ctrl Pts',(-2.73012016971229,-12.275251859102,129.248944868544)) ;
#11863=CARTESIAN_POINT('Ctrl Pts',(-2.73373233104272,-12.2676382180192,
129.264677387526)) ;
#11864=CARTESIAN_POINT('Ctrl Pts',(-2.73692362652984,-12.2586944860079,
129.279683128273)) ;
#11865=CARTESIAN_POINT('Ctrl Pts',(-2.73963424355121,-12.2510978744367,
129.292428678302)) ;
#11866=CARTESIAN_POINT('Ctrl Pts',(-2.74204130819701,-12.2425426265771,
129.304650128334)) ;
#11867=CARTESIAN_POINT('Ctrl Pts',(-2.74416631789832,-12.2331361681733,
129.316199440896)) ;
#11868=CARTESIAN_POINT('Ctrl Pts',(-2.74722389952739,-12.2196016349464,
129.332817231345)) ;
#11869=CARTESIAN_POINT('Ctrl Pts',(-2.7497090908537,-12.2042764178469,129.348077230942)) ;
#11870=CARTESIAN_POINT('Ctrl Pts',(-2.75171298541311,-12.1874596100186,
129.361617491048)) ;
#11871=CARTESIAN_POINT('Ctrl Pts',(-2.75231427877979,-12.1824135186719,
129.365680413693)) ;
#11872=CARTESIAN_POINT('Ctrl Pts',(-2.75287230997023,-12.1772334001408,
129.369588707344)) ;
#11873=CARTESIAN_POINT('Ctrl Pts',(-2.75338972338882,-12.1719280645935,
129.373333128882)) ;
#11874=CARTESIAN_POINT('Ctrl Pts',(-2.75478034225058,-12.1576692544915,
129.383396770507)) ;
#11875=CARTESIAN_POINT('Ctrl Pts',(-2.75587337962017,-12.1425172907069,
129.392264479144)) ;
#11876=CARTESIAN_POINT('Ctrl Pts',(-2.75673073612266,-12.126702243247,129.399759564773)) ;
#11877=CARTESIAN_POINT('Ctrl Pts',(-2.7575867422374,-12.1109121054322,129.407242845194)) ;
#11878=CARTESIAN_POINT('Ctrl Pts',(-2.75820769589563,-12.094461586077,129.413357491779)) ;
#11879=CARTESIAN_POINT('Ctrl Pts',(-2.75866992540113,-12.0776047742543,
129.417970647894)) ;
#11880=CARTESIAN_POINT('Ctrl Pts',(-2.75881852718141,-12.0721854918048,
129.419453727627)) ;
#11881=CARTESIAN_POINT('Ctrl Pts',(-2.75895084447806,-12.066724371869,129.420781972381)) ;
#11882=CARTESIAN_POINT('Ctrl Pts',(-2.75906976307799,-12.0612302416584,
129.421951988857)) ;
#11883=CARTESIAN_POINT('Ctrl Pts',(-2.75943121665534,-12.0445308101116,
129.425508258785)) ;
#11884=CARTESIAN_POINT('Ctrl Pts',(-2.75966668090157,-12.0275399677879,
129.427596283874)) ;
#11885=CARTESIAN_POINT('Ctrl Pts',(-2.75973265423389,-12.0105187380521,
129.428204893541)) ;
#11886=CARTESIAN_POINT('Ctrl Pts',(-2.75974625769244,-12.0070090230641,
129.428330386616)) ;
#11887=CARTESIAN_POINT('Ctrl Pts',(-2.75975271216325,-12.0034980264116,
129.428393146724)) ;
#11888=CARTESIAN_POINT('Ctrl Pts',(-2.759751725504,-11.9999880414369,129.428393336592)) ;
#11889=CARTESIAN_POINT('Ctrl Pts',(-2.75974584112683,-11.9790546995273,
129.428394468955)) ;
#11890=CARTESIAN_POINT('Ctrl Pts',(-2.75947403180639,-11.9581302988716,
129.426166401703)) ;
#11891=CARTESIAN_POINT('Ctrl Pts',(-2.75902641398435,-11.9376174897222,
129.421710411074)) ;
#11892=CARTESIAN_POINT('Ctrl Pts',(-2.75866386022208,-11.9210028784051,
129.418101224648)) ;
#11893=CARTESIAN_POINT('Ctrl Pts',(-2.75818766763213,-11.9046908809968,
129.413035393923)) ;
#11894=CARTESIAN_POINT('Ctrl Pts',(-2.75751170425596,-11.8889291444235,
129.406626935435)) ;
#11895=CARTESIAN_POINT('Ctrl Pts',(-2.75683470809671,-11.873143325991,129.400208685665)) ;
#11896=CARTESIAN_POINT('Ctrl Pts',(-2.75595743654763,-11.8579101505729,
129.392444012836)) ;
#11897=CARTESIAN_POINT('Ctrl Pts',(-2.75480870069275,-11.8434563528919,
129.383492264161)) ;
#11898=CARTESIAN_POINT('Ctrl Pts',(-2.75439405639888,-11.8382391528647,
129.380261067456)) ;
#11899=CARTESIAN_POINT('Ctrl Pts',(-2.75394417936731,-11.833123239302,129.376875604947)) ;
#11900=CARTESIAN_POINT('Ctrl Pts',(-2.75345616280295,-11.8281183129539,
129.373344659306)) ;
#11901=CARTESIAN_POINT('Ctrl Pts',(-2.75206020747337,-11.8138018857667,
129.363244505446)) ;
#11902=CARTESIAN_POINT('Ctrl Pts',(-2.75033870662451,-11.8003405868789,
129.351914598047)) ;
#11903=CARTESIAN_POINT('Ctrl Pts',(-2.74825336831493,-11.7879525678663,
129.339545138952)) ;
#11904=CARTESIAN_POINT('Ctrl Pts',(-2.74617111060459,-11.7755828492521,
129.327193952837)) ;
#11905=CARTESIAN_POINT('Ctrl Pts',(-2.74372623641133,-11.7642837734984,
129.313806712992)) ;
#11906=CARTESIAN_POINT('Ctrl Pts',(-2.74089327437816,-11.7542382902871,
129.299609736567)) ;
#11907=CARTESIAN_POINT('Ctrl Pts',(-2.7380631545389,-11.7442028852945,129.285427003382)) ;
#11908=CARTESIAN_POINT('Ctrl Pts',(-2.73484590441089,-11.7354189851583,
129.270436681145)) ;
#11909=CARTESIAN_POINT('Ctrl Pts',(-2.73122631627443,-11.7280275951829,
129.25489416535)) ;
#11910=CARTESIAN_POINT('Ctrl Pts',(-2.72760713631055,-11.7206370387174,
129.239353402248)) ;
#11911=CARTESIAN_POINT('Ctrl Pts',(-2.72358591267336,-11.7146389846951,
129.223261164881)) ;
#11912=CARTESIAN_POINT('Ctrl Pts',(-2.71915475623112,-11.7101274659389,
129.206894126674)) ;
#11913=CARTESIAN_POINT('Ctrl Pts',(-2.71745866047623,-11.7084006102274,
129.200629381932)) ;
#11914=CARTESIAN_POINT('Ctrl Pts',(-2.71570256550788,-11.7068910343395,
129.194324551297)) ;
#11915=CARTESIAN_POINT('Ctrl Pts',(-2.71388621274829,-11.7056020706594,
129.187995687355)) ;
#11916=CARTESIAN_POINT('Ctrl Pts',(-2.70967040184253,-11.702610346111,129.173306198496)) ;
#11917=CARTESIAN_POINT('Ctrl Pts',(-2.70513486121312,-11.7008139286664,
129.158501522976)) ;
#11918=CARTESIAN_POINT('Ctrl Pts',(-2.70028788857756,-11.7002205909573,
129.143816064066)) ;
#11919=CARTESIAN_POINT('Ctrl Pts',(-2.69908743359452,-11.7000736383617,
129.14017890049)) ;
#11920=CARTESIAN_POINT('Ctrl Pts',(-2.69786787424697,-11.7000002331707,
129.136549047369)) ;
#11921=CARTESIAN_POINT('Ctrl Pts',(-2.6966293264623,-11.7000000005548,129.132930036242)) ;
#11922=CARTESIAN_POINT('Ctrl Pts',(-2.69662735734983,-11.7000000001849,
129.132924282535)) ;
#11923=CARTESIAN_POINT('Ctrl Pts',(-2.6966253881834,-11.7,129.132918528839)) ;
#11924=CARTESIAN_POINT('Ctrl Pts',(-2.69662341896302,-11.7,129.132912775153)) ;
#11925=CARTESIAN_POINT('',(2.69661245380302,-11.7,130.979127236674)) ;
#11926=CARTESIAN_POINT('',(-5.63784594017984E-6,-11.7,130.056019952763)) ;
#11927=CARTESIAN_POINT('',(2.69638403966492,-12.3,130.979049045863)) ;
#11928=CARTESIAN_POINT('Ctrl Pts',(2.69661245380302,-11.7,130.979127236674)) ;
#11929=CARTESIAN_POINT('Ctrl Pts',(2.69113431078088,-11.7,130.995132749034)) ;
#11930=CARTESIAN_POINT('Ctrl Pts',(2.68523850579487,-11.7014358277356,131.011061288262)) ;
#11931=CARTESIAN_POINT('Ctrl Pts',(2.67909713495093,-11.7043096952124,131.026685859201)) ;
#11932=CARTESIAN_POINT('Ctrl Pts',(2.67315243899305,-11.7070915282602,131.041810059655)) ;
#11933=CARTESIAN_POINT('Ctrl Pts',(2.66697792645336,-11.7112204554927,131.056648651996)) ;
#11934=CARTESIAN_POINT('Ctrl Pts',(2.66072866461214,-11.7166458361922,131.070998734394)) ;
#11935=CARTESIAN_POINT('Ctrl Pts',(2.65416927601188,-11.7223404576078,131.086060956027)) ;
#11936=CARTESIAN_POINT('Ctrl Pts',(2.64752788465194,-11.7294635845994,131.100583957441)) ;
#11937=CARTESIAN_POINT('Ctrl Pts',(2.64097785752022,-11.7378976704316,131.114350489788)) ;
#11938=CARTESIAN_POINT('Ctrl Pts',(2.63442783038849,-11.7463317562638,131.128117022136)) ;
#11939=CARTESIAN_POINT('Ctrl Pts',(2.62796945565154,-11.7560762459643,131.141126243614)) ;
#11940=CARTESIAN_POINT('Ctrl Pts',(2.62176544834925,-11.7669595581195,131.153192022274)) ;
#11941=CARTESIAN_POINT('Ctrl Pts',(2.6152474940389,-11.7783936083899,131.165868376475)) ;
#11942=CARTESIAN_POINT('Ctrl Pts',(2.60900474534324,-11.7910966245474,131.177519621961)) ;
#11943=CARTESIAN_POINT('Ctrl Pts',(2.60320587339938,-11.8048541799202,131.187988390373)) ;
#11944=CARTESIAN_POINT('Ctrl Pts',(2.6000608605201,-11.8123155774565,131.193666117318)) ;
#11945=CARTESIAN_POINT('Ctrl Pts',(2.59704619393286,-11.8200865437393,131.19899666061)) ;
#11946=CARTESIAN_POINT('Ctrl Pts',(2.59418713529822,-11.8281289649774,131.203959724246)) ;
#11947=CARTESIAN_POINT('Ctrl Pts',(2.5892779034638,-11.8419384440448,131.212481700571)) ;
#11948=CARTESIAN_POINT('Ctrl Pts',(2.584817673955,-11.8565971445557,131.219948801914)) ;
#11949=CARTESIAN_POINT('Ctrl Pts',(2.58096540364702,-11.8718908385621,131.2262640739)) ;
#11950=CARTESIAN_POINT('Ctrl Pts',(2.57711829862176,-11.8871640261537,131.232570878109)) ;
#11951=CARTESIAN_POINT('Ctrl Pts',(2.57387765122074,-11.903069835983,131.237728566734)) ;
#11952=CARTESIAN_POINT('Ctrl Pts',(2.57138717998916,-11.9193690965159,131.24168322434)) ;
#11953=CARTESIAN_POINT('Ctrl Pts',(2.57046502112798,-11.9254043027614,131.243147534591)) ;
#11954=CARTESIAN_POINT('Ctrl Pts',(2.56964556070338,-11.9314932494922,131.244447352992)) ;
#11955=CARTESIAN_POINT('Ctrl Pts',(2.56893554017386,-11.9376231925806,131.245581562453)) ;
#11956=CARTESIAN_POINT('Ctrl Pts',(2.5665594885193,-11.9581367704451,131.249377143222)) ;
#11957=CARTESIAN_POINT('Ctrl Pts',(2.56541360463764,-11.979054438517,131.251304739745)) ;
#11958=CARTESIAN_POINT('Ctrl Pts',(2.56541995514723,-11.9999847393984,131.251308039005)) ;
#11959=CARTESIAN_POINT('Ctrl Pts',(2.56542503678568,-12.0167330365428,131.251310679052)) ;
#11960=CARTESIAN_POINT('Ctrl Pts',(2.56616861398396,-12.0335095446092,131.250079103225)) ;
#11961=CARTESIAN_POINT('Ctrl Pts',(2.56768297526068,-12.0500600292145,131.247636932901)) ;
#11962=CARTESIAN_POINT('Ctrl Pts',(2.56802487089586,-12.0537966134323,131.247085566865)) ;
#11963=CARTESIAN_POINT('Ctrl Pts',(2.56840598653394,-12.0575216852744,131.246472693794)) ;
#11964=CARTESIAN_POINT('Ctrl Pts',(2.5688265749632,-12.061232350046,131.245798932508)) ;
#11965=CARTESIAN_POINT('Ctrl Pts',(2.57077173436107,-12.078393626845,131.242682886019)) ;
#11966=CARTESIAN_POINT('Ctrl Pts',(2.57356133844419,-12.0952290052352,131.238264044836)) ;
#11967=CARTESIAN_POINT('Ctrl Pts',(2.57705639028525,-12.1114767204747,131.232586883274)) ;
#11968=CARTESIAN_POINT('Ctrl Pts',(2.58055813602547,-12.1277555541559,131.226898848526)) ;
#11969=CARTESIAN_POINT('Ctrl Pts',(2.58476793490904,-12.1434438420947,131.219947959217)) ;
#11970=CARTESIAN_POINT('Ctrl Pts',(2.58953071272326,-12.1583008404025,131.211823573806)) ;
#11971=CARTESIAN_POINT('Ctrl Pts',(2.5910131951914,-12.1629252928501,131.209294743068)) ;
#11972=CARTESIAN_POINT('Ctrl Pts',(2.59254914837815,-12.1674694062319,131.206652524045)) ;
#11973=CARTESIAN_POINT('Ctrl Pts',(2.5941336213501,-12.1719265063663,131.203900413003)) ;
#11974=CARTESIAN_POINT('Ctrl Pts',(2.59998807347437,-12.188394997664,131.193731667545)) ;
#11975=CARTESIAN_POINT('Ctrl Pts',(2.60650465511311,-12.2036678470003,131.182063449917)) ;
#11976=CARTESIAN_POINT('Ctrl Pts',(2.61344658327035,-12.2174761624351,131.169080221189)) ;
#11977=CARTESIAN_POINT('Ctrl Pts',(2.62038683170025,-12.2312811366937,131.156100133992)) ;
#11978=CARTESIAN_POINT('Ctrl Pts',(2.62775218527328,-12.2436222312856,131.141805775879)) ;
#11979=CARTESIAN_POINT('Ctrl Pts',(2.63529483228866,-12.2542695739186,131.126414193534)) ;
#11980=CARTESIAN_POINT('Ctrl Pts',(2.6427400745756,-12.2647794182018,131.111221376012)) ;
#11981=CARTESIAN_POINT('Ctrl Pts',(2.65035803048437,-12.2736388840425,131.094959578602)) ;
#11982=CARTESIAN_POINT('Ctrl Pts',(2.65789995579973,-12.2806656473848,131.077867956574)) ;
#11983=CARTESIAN_POINT('Ctrl Pts',(2.66251197593969,-12.2849626369064,131.06741612873)) ;
#11984=CARTESIAN_POINT('Ctrl Pts',(2.66709536320241,-12.2885750329263,131.056654571847)) ;
#11985=CARTESIAN_POINT('Ctrl Pts',(2.6715913359282,-12.2914688040928,131.045643523228)) ;
#11986=CARTESIAN_POINT('Ctrl Pts',(2.67746084722523,-12.2952466345178,131.03126855296)) ;
#11987=CARTESIAN_POINT('Ctrl Pts',(2.68317659539627,-12.2977926378117,131.016482324032)) ;
#11988=CARTESIAN_POINT('Ctrl Pts',(2.68858815040895,-12.299058953697,131.001476237306)) ;
#11989=CARTESIAN_POINT('Ctrl Pts',(2.6912675760568,-12.2996859452462,130.99404626689)) ;
#11990=CARTESIAN_POINT('Ctrl Pts',(2.69387236298024,-12.3,130.986562585859)) ;
#11991=CARTESIAN_POINT('Ctrl Pts',(2.69638403966493,-12.3,130.979049045863)) ;
#11992=CARTESIAN_POINT('Ctrl Pts',(2.69638403966492,-12.3,130.979049045863)) ;
#11993=CARTESIAN_POINT('Ctrl Pts',(2.70225022747721,-12.3,130.962308165737)) ;
#11994=CARTESIAN_POINT('Ctrl Pts',(2.70764519706473,-12.2984224104787,130.945430926132)) ;
#11995=CARTESIAN_POINT('Ctrl Pts',(2.71258182346257,-12.2953054737208,130.928717527059)) ;
#11996=CARTESIAN_POINT('Ctrl Pts',(2.71752666370191,-12.2921833508252,130.911976319276)) ;
#11997=CARTESIAN_POINT('Ctrl Pts',(2.72201142529684,-12.2875169592251,130.895400108087)) ;
#11998=CARTESIAN_POINT('Ctrl Pts',(2.72605366680566,-12.2813952242403,130.879277100824)) ;
#11999=CARTESIAN_POINT('Ctrl Pts',(2.73011297470477,-12.2752476432197,130.863086022039)) ;
#12000=CARTESIAN_POINT('Ctrl Pts',(2.73372582255887,-12.267632716394,130.847352552993)) ;
#12001=CARTESIAN_POINT('Ctrl Pts',(2.736917703741,-12.2586875021641,130.832346039818)) ;
#12002=CARTESIAN_POINT('Ctrl Pts',(2.7396281801801,-12.2510914197822,130.819602833517)) ;
#12003=CARTESIAN_POINT('Ctrl Pts',(2.74203517470168,-12.242537011286,130.807383607764)) ;
#12004=CARTESIAN_POINT('Ctrl Pts',(2.74416011607381,-12.2331316461142,130.795836299742)) ;
#12005=CARTESIAN_POINT('Ctrl Pts',(2.7472186064759,-12.2195942283374,130.779215920836)) ;
#12006=CARTESIAN_POINT('Ctrl Pts',(2.74970433309686,-12.2042654698107,130.763953772354)) ;
#12007=CARTESIAN_POINT('Ctrl Pts',(2.75170825078127,-12.1874445705517,130.750411931767)) ;
#12008=CARTESIAN_POINT('Ctrl Pts',(2.75230902884218,-12.1824016352464,130.746352064042)) ;
#12009=CARTESIAN_POINT('Ctrl Pts',(2.75286657377173,-12.1772248561933,130.742446608027)) ;
#12010=CARTESIAN_POINT('Ctrl Pts',(2.75338351917669,-12.1719230237542,130.738704786761)) ;
#12011=CARTESIAN_POINT('Ctrl Pts',(2.75477436360932,-12.1576584146486,130.72863739623)) ;
#12012=CARTESIAN_POINT('Ctrl Pts',(2.75586710296249,-12.1425000310335,130.719766833699)) ;
#12013=CARTESIAN_POINT('Ctrl Pts',(2.75672435039289,-12.1266781224806,130.712270137096)) ;
#12014=CARTESIAN_POINT('Ctrl Pts',(2.75758023008551,-12.1108814577735,130.704785401468)) ;
#12015=CARTESIAN_POINT('Ctrl Pts',(2.75820125540657,-12.0944239978118,130.698670482248)) ;
#12016=CARTESIAN_POINT('Ctrl Pts',(2.75866445797828,-12.0775600039634,130.694058577431)) ;
#12017=CARTESIAN_POINT('Ctrl Pts',(2.75880226333131,-12.072542871573,130.692686509981)) ;
#12018=CARTESIAN_POINT('Ctrl Pts',(2.75892620482364,-12.0674898913635,130.691447167072)) ;
#12019=CARTESIAN_POINT('Ctrl Pts',(2.7590385826833,-12.0624080592774,130.690343262022)) ;
#12020=CARTESIAN_POINT('Ctrl Pts',(2.7594077366967,-12.0457145689792,130.686717005206)) ;
#12021=CARTESIAN_POINT('Ctrl Pts',(2.75964985448609,-12.0287234593521,130.684558819819)) ;
#12022=CARTESIAN_POINT('Ctrl Pts',(2.75972259697515,-12.0116958892487,130.683881526958)) ;
#12023=CARTESIAN_POINT('Ctrl Pts',(2.75973926506155,-12.0077942216904,130.68372633326)) ;
#12024=CARTESIAN_POINT('Ctrl Pts',(2.75974711015346,-12.0038906537072,130.683648688519)) ;
#12025=CARTESIAN_POINT('Ctrl Pts',(2.75974574765666,-11.99998833549,130.683648382481)) ;
#12026=CARTESIAN_POINT('Ctrl Pts',(2.75973857892329,-11.9794564129564,130.683646772273)) ;
#12027=CARTESIAN_POINT('Ctrl Pts',(2.7594754211691,-11.9589331107215,130.685789331442)) ;
#12028=CARTESIAN_POINT('Ctrl Pts',(2.75904489406721,-11.9387965376136,130.690077363479)) ;
#12029=CARTESIAN_POINT('Ctrl Pts',(2.75868965035837,-11.9221811122835,130.69361557605)) ;
#12030=CARTESIAN_POINT('Ctrl Pts',(2.7582220316112,-11.9058614188827,130.69860992392)) ;
#12031=CARTESIAN_POINT('Ctrl Pts',(2.75755623473998,-11.8900851853341,130.704948007217)) ;
#12032=CARTESIAN_POINT('Ctrl Pts',(2.75688942885809,-11.8742850430101,130.711295695837)) ;
#12033=CARTESIAN_POINT('Ctrl Pts',(2.75602394875841,-11.8590307121269,130.718990888978)) ;
#12034=CARTESIAN_POINT('Ctrl Pts',(2.75488898277129,-11.84454928171,130.727875740134)) ;
#12035=CARTESIAN_POINT('Ctrl Pts',(2.75445028470273,-11.8389517786781,130.731309999033)) ;
#12036=CARTESIAN_POINT('Ctrl Pts',(2.75397147789854,-11.8334694651347,130.734921549577)) ;
#12037=CARTESIAN_POINT('Ctrl Pts',(2.75344902648665,-11.8281142579715,130.738699659381)) ;
#12038=CARTESIAN_POINT('Ctrl Pts',(2.75205230124255,-11.8137976098355,130.748800084451)) ;
#12039=CARTESIAN_POINT('Ctrl Pts',(2.75033014856981,-11.8003361745224,130.76013034769)) ;
#12040=CARTESIAN_POINT('Ctrl Pts',(2.74824424245493,-11.7879481058189,130.77250021509)) ;
#12041=CARTESIAN_POINT('Ctrl Pts',(2.74616141622784,-11.7755783283804,130.7848518181)) ;
#12042=CARTESIAN_POINT('Ctrl Pts',(2.74371605674675,-11.7642792817948,130.7982395287)) ;
#12043=CARTESIAN_POINT('Ctrl Pts',(2.74088265796537,-11.7542339159119,130.812436999292)) ;
#12044=CARTESIAN_POINT('Ctrl Pts',(2.73805210114096,-11.7441986257365,130.82662022953)) ;
#12045=CARTESIAN_POINT('Ctrl Pts',(2.73483446227555,-11.7354149289329,130.841611072598)) ;
#12046=CARTESIAN_POINT('Ctrl Pts',(2.73121449845122,-11.7280238296724,130.857154104223)) ;
#12047=CARTESIAN_POINT('Ctrl Pts',(2.72759494388778,-11.7206335660247,130.872695378606)) ;
#12048=CARTESIAN_POINT('Ctrl Pts',(2.72357335891403,-11.7146358913333,130.888788121982)) ;
#12049=CARTESIAN_POINT('Ctrl Pts',(2.71914181881838,-11.7101248366017,130.905155633563)) ;
#12050=CARTESIAN_POINT('Ctrl Pts',(2.71744585098747,-11.7083984382067,130.911419544645)) ;
#12051=CARTESIAN_POINT('Ctrl Pts',(2.71568990011048,-11.7068892616191,130.917723523857)) ;
#12052=CARTESIAN_POINT('Ctrl Pts',(2.71387370572788,-11.7056006375845,130.924051524917)) ;
#12053=CARTESIAN_POINT('Ctrl Pts',(2.70965766191582,-11.7026092752947,130.938741103285)) ;
#12054=CARTESIAN_POINT('Ctrl Pts',(2.70512187378689,-11.7008132376122,130.953545840774)) ;
#12055=CARTESIAN_POINT('Ctrl Pts',(2.70027461522219,-11.7002202946038,130.968231324017)) ;
#12056=CARTESIAN_POINT('Ctrl Pts',(2.69907513223611,-11.7000735673267,130.971865334264)) ;
#12057=CARTESIAN_POINT('Ctrl Pts',(2.69785657570499,-11.700000260626,130.975492044451)) ;
#12058=CARTESIAN_POINT('Ctrl Pts',(2.69661906089626,-11.7000000006939,130.979107932074)) ;
#12059=CARTESIAN_POINT('Ctrl Pts',(2.69661685859934,-11.7000000002313,130.979114366953)) ;
#12060=CARTESIAN_POINT('Ctrl Pts',(2.69661465623493,-11.7,130.97912080182)) ;
#12061=CARTESIAN_POINT('Ctrl Pts',(2.69661245380302,-11.7,130.979127236674)) ;
#12062=CARTESIAN_POINT('Ctrl Pts',(-2.69662341896302,-11.7,129.132912775153)) ;
#12063=CARTESIAN_POINT('Ctrl Pts',(-2.69114835812364,-11.7,129.116915692321)) ;
#12064=CARTESIAN_POINT('Ctrl Pts',(-2.68525611727231,-11.7014343001684,
129.100995500579)) ;
#12065=CARTESIAN_POINT('Ctrl Pts',(-2.67911851841346,-11.704305115768,129.085378841304)) ;
#12066=CARTESIAN_POINT('Ctrl Pts',(-2.67317444510001,-11.7070854112526,
129.070254593244)) ;
#12067=CARTESIAN_POINT('Ctrl Pts',(-2.66700051540259,-11.7112127500097,
129.055415834658)) ;
#12068=CARTESIAN_POINT('Ctrl Pts',(-2.66075178708574,-11.7166365107268,
129.041065462901)) ;
#12069=CARTESIAN_POINT('Ctrl Pts',(-2.6541978921369,-11.7223251494649,129.026014267809)) ;
#12070=CARTESIAN_POINT('Ctrl Pts',(-2.64756206239371,-11.7294401036985,
129.01150134337)) ;
#12071=CARTESIAN_POINT('Ctrl Pts',(-2.6410172671884,-11.7378641349517,128.997743455817)) ;
#12072=CARTESIAN_POINT('Ctrl Pts',(-2.6344724719831,-11.746288166205,128.983985568265)) ;
#12073=CARTESIAN_POINT('Ctrl Pts',(-2.6280189984544,-11.7560207217575,128.970983556401)) ;
#12074=CARTESIAN_POINT('Ctrl Pts',(-2.62181919984631,-11.7668906835074,
128.958923174318)) ;
#12075=CARTESIAN_POINT('Ctrl Pts',(-2.61529979661753,-11.7783210005563,
128.946241069807)) ;
#12076=CARTESIAN_POINT('Ctrl Pts',(-2.60905533324604,-11.7910209995357,
128.93458392869)) ;
#12077=CARTESIAN_POINT('Ctrl Pts',(-2.60325456376142,-11.8047762867985,
128.924109243443)) ;
#12078=CARTESIAN_POINT('Ctrl Pts',(-2.6000985336779,-11.8122601388157,128.918410271636)) ;
#12079=CARTESIAN_POINT('Ctrl Pts',(-2.59707362546236,-11.8200557510676,
128.913060687359)) ;
#12080=CARTESIAN_POINT('Ctrl Pts',(-2.59420535418644,-11.8281246442548,
128.908080996712)) ;
#12081=CARTESIAN_POINT('Ctrl Pts',(-2.5893020251905,-11.8419184713108,128.899568182132)) ;
#12082=CARTESIAN_POINT('Ctrl Pts',(-2.58484664609052,-11.8565598978575,
128.892107698161)) ;
#12083=CARTESIAN_POINT('Ctrl Pts',(-2.58099731417302,-11.8718351673646,
128.885796564058)) ;
#12084=CARTESIAN_POINT('Ctrl Pts',(-2.57715299184827,-11.8870905573495,
128.879493643383)) ;
#12085=CARTESIAN_POINT('Ctrl Pts',(-2.57391326831685,-11.9029774700525,
128.874337456948)) ;
#12086=CARTESIAN_POINT('Ctrl Pts',(-2.57142102170537,-11.9192571844022,
128.87038198769)) ;
#12087=CARTESIAN_POINT('Ctrl Pts',(-2.57043225798016,-11.9257159316753,
128.868812710998)) ;
#12088=CARTESIAN_POINT('Ctrl Pts',(-2.5695609749712,-11.9322362762841,128.867431924904)) ;
#12089=CARTESIAN_POINT('Ctrl Pts',(-2.56881539891482,-11.9388025611347,
128.866240967448)) ;
#12090=CARTESIAN_POINT('Ctrl Pts',(-2.56652889617113,-11.958939780132,128.862588586892)) ;
#12091=CARTESIAN_POINT('Ctrl Pts',(-2.56542885216133,-11.979456219035,128.860733766742)) ;
#12092=CARTESIAN_POINT('Ctrl Pts',(-2.56543663567068,-11.9999849854663,
128.860730016324)) ;
#12093=CARTESIAN_POINT('Ctrl Pts',(-2.56544298788344,-12.0167387511885,
128.860726955564)) ;
#12094=CARTESIAN_POINT('Ctrl Pts',(-2.5661879677875,-12.0335208418553,128.861959033802)) ;
#12095=CARTESIAN_POINT('Ctrl Pts',(-2.5677025541412,-12.0500768655049,128.864403142488)) ;
#12096=CARTESIAN_POINT('Ctrl Pts',(-2.5680800528906,-12.0542033243281,128.865012317376)) ;
#12097=CARTESIAN_POINT('Ctrl Pts',(-2.56850527884464,-12.0583157490876,
128.865696546005)) ;
#12098=CARTESIAN_POINT('Ctrl Pts',(-2.56897854879208,-12.0624102439602,
128.866454994808)) ;
#12099=CARTESIAN_POINT('Ctrl Pts',(-2.57096162074754,-12.0795667906575,
128.869633008879)) ;
#12100=CARTESIAN_POINT('Ctrl Pts',(-2.5737883114194,-12.0963905502262,128.87411440536)) ;
#12101=CARTESIAN_POINT('Ctrl Pts',(-2.57731833127862,-12.1126199097541,
128.879853721937)) ;
#12102=CARTESIAN_POINT('Ctrl Pts',(-2.58085515675867,-12.1288805583034,
128.885604103498)) ;
#12103=CARTESIAN_POINT('Ctrl Pts',(-2.58509792556663,-12.1445438865275,
128.89261696687)) ;
#12104=CARTESIAN_POINT('Ctrl Pts',(-2.58989029851729,-12.1593695433182,
128.900802076266)) ;
#12105=CARTESIAN_POINT('Ctrl Pts',(-2.59126556748867,-12.1636240673243,
128.903150960023)) ;
#12106=CARTESIAN_POINT('Ctrl Pts',(-2.59268600730169,-12.1678097827635,
128.905596117215)) ;
#12107=CARTESIAN_POINT('Ctrl Pts',(-2.59414771277222,-12.1719214624428,
128.908134800458)) ;
#12108=CARTESIAN_POINT('Ctrl Pts',(-2.60000316994638,-12.1883924716587,
128.918304531167)) ;
#12109=CARTESIAN_POINT('Ctrl Pts',(-2.60652054073974,-12.2036674715057,
128.929974259017)) ;
#12110=CARTESIAN_POINT('Ctrl Pts',(-2.61346311317316,-12.2174775116136,
128.942959386473)) ;
#12111=CARTESIAN_POINT('Ctrl Pts',(-2.6204040657376,-12.2312843295072,128.955941484188)) ;
#12112=CARTESIAN_POINT('Ctrl Pts',(-2.62776998615462,-12.2436268175001,
128.970238264367)) ;
#12113=CARTESIAN_POINT('Ctrl Pts',(-2.63531313020966,-12.2542750466656,
128.985632546937)) ;
#12114=CARTESIAN_POINT('Ctrl Pts',(-2.64275872104803,-12.2647855654813,
129.000827739874)) ;
#12115=CARTESIAN_POINT('Ctrl Pts',(-2.65037695111223,-12.2736452755129,
129.017092143517)) ;
#12116=CARTESIAN_POINT('Ctrl Pts',(-2.65791915501401,-12.2806718082327,
129.034186487092)) ;
#12117=CARTESIAN_POINT('Ctrl Pts',(-2.66252943392023,-12.2849668758288,
129.044635646598)) ;
#12118=CARTESIAN_POINT('Ctrl Pts',(-2.66711110523052,-12.2885777401896,
129.055394321234)) ;
#12119=CARTESIAN_POINT('Ctrl Pts',(-2.67160547807788,-12.29147039969,129.066402321398)) ;
#12120=CARTESIAN_POINT('Ctrl Pts',(-2.67747472379133,-12.2952479521871,
129.080777777099)) ;
#12121=CARTESIAN_POINT('Ctrl Pts',(-2.68319031030512,-12.2977936307649,
129.095564468109)) ;
#12122=CARTESIAN_POINT('Ctrl Pts',(-2.68860188327558,-12.2990595646063,
129.110570961495)) ;
#12123=CARTESIAN_POINT('Ctrl Pts',(-2.69128038443391,-12.2996861486475,
129.11799854496)) ;
#12124=CARTESIAN_POINT('Ctrl Pts',(-2.69388434284319,-12.3,129.125479787993)) ;
#12125=CARTESIAN_POINT('Ctrl Pts',(-2.69639531535756,-12.3,129.132990859662)) ;
#12126=CARTESIAN_POINT('Ctrl Pts',(-2.69634333633521,12.2999450599054,129.133008652785)) ;
#12127=CARTESIAN_POINT('Ctrl Pts',(-2.66564577776436,12.301084845338,129.041173414331)) ;
#12128=CARTESIAN_POINT('Ctrl Pts',(-2.60382900342522,12.229363413126,128.921431450579)) ;
#12129=CARTESIAN_POINT('Ctrl Pts',(-2.56885602948563,12.0820021895678,128.86657194469)) ;
#12130=CARTESIAN_POINT('Ctrl Pts',(-2.56422288068699,12.0003596690755,128.858780178468)) ;
#12131=CARTESIAN_POINT('Ctrl Pts',(-2.56880156245784,11.9185468804347,128.866672863108)) ;
#12132=CARTESIAN_POINT('Ctrl Pts',(-2.60359744333516,11.7703554429164,128.920157345138)) ;
#12133=CARTESIAN_POINT('Ctrl Pts',(-2.70921355792956,11.6499856574159,129.128497465002)) ;
#12134=CARTESIAN_POINT('Ctrl Pts',(-2.75358463094391,11.7702822363656,129.358212195121)) ;
#12135=CARTESIAN_POINT('Ctrl Pts',(-2.75873449232472,11.918576320469,129.421574629153)) ;
#12136=CARTESIAN_POINT('Ctrl Pts',(-2.75999748629359,11.9999479462354,129.430655077509)) ;
#12137=CARTESIAN_POINT('Ctrl Pts',(-2.75887443013528,12.0816127336495,129.421791811517)) ;
#12138=CARTESIAN_POINT('Ctrl Pts',(-2.75297468183829,12.2291419145039,129.357308950944)) ;
#12139=CARTESIAN_POINT('Ctrl Pts',(-2.7283570304801,12.301091767988,129.224375795964)) ;
#12140=CARTESIAN_POINT('Ctrl Pts',(-2.69634333633521,12.2999450599054,129.133008652785)) ;
#12141=CARTESIAN_POINT('Ctrl Pts',(-2.83831085827015,12.4500000000046,129.084411247894)) ;
#12142=CARTESIAN_POINT('Ctrl Pts',(-2.78948214878003,12.4517099925444,128.939496819705)) ;
#12143=CARTESIAN_POINT('Ctrl Pts',(-2.70167351947378,12.3441081369419,128.747029727252)) ;
#12144=CARTESIAN_POINT('Ctrl Pts',(-2.65407477200972,12.1230258146196,128.657777998572)) ;
#12145=CARTESIAN_POINT('Ctrl Pts',(-2.64768441549552,12.0005396024158,128.645155374403)) ;
#12146=CARTESIAN_POINT('Ctrl Pts',(-2.65403071331193,11.8777979413041,128.657923013224)) ;
#12147=CARTESIAN_POINT('Ctrl Pts',(-2.70121137800042,11.6554700696645,128.745050570368)) ;
#12148=CARTESIAN_POINT('Ctrl Pts',(-2.85184170514048,11.4748823176714,129.079612830176)) ;
#12149=CARTESIAN_POINT('Ctrl Pts',(-2.93806835347429,11.6553602398041,129.43686799927)) ;
#12150=CARTESIAN_POINT('Ctrl Pts',(-2.95399843334428,11.8778421094138,129.534266097453)) ;
#12151=CARTESIAN_POINT('Ctrl Pts',(-2.95686297599919,11.9999219050466,129.548308897304)) ;
#12152=CARTESIAN_POINT('Ctrl Pts',(-2.9541885151246,12.1224415237254,129.534619673828)) ;
#12153=CARTESIAN_POINT('Ctrl Pts',(-2.93724684308448,12.3437758281832,129.435392991623)) ;
#12154=CARTESIAN_POINT('Ctrl Pts',(-2.88852216719596,12.4517203783323,129.228824659478)) ;
#12155=CARTESIAN_POINT('Ctrl Pts',(-2.83831085827015,12.4500000000046,129.084411247894)) ;
#12156=CARTESIAN_POINT('',(-2.83831085827015,12.4500000000046,129.084411247894)) ;
#12157=CARTESIAN_POINT('',(-2.69639531535756,12.3,129.132990859662)) ;
#12158=CARTESIAN_POINT('Ctrl Pts',(-2.83831085827015,12.4500000000046,129.084411247894)) ;
#12159=CARTESIAN_POINT('Ctrl Pts',(-2.78948214878003,12.4517099925444,128.939496819705)) ;
#12160=CARTESIAN_POINT('Ctrl Pts',(-2.70167351947378,12.3441081369419,128.747029727252)) ;
#12161=CARTESIAN_POINT('Ctrl Pts',(-2.65407477200972,12.1230258146196,128.657777998572)) ;
#12162=CARTESIAN_POINT('Ctrl Pts',(-2.64768441549552,12.0005396024158,128.645155374403)) ;
#12163=CARTESIAN_POINT('Ctrl Pts',(-2.65403071331193,11.8777979413041,128.657923013224)) ;
#12164=CARTESIAN_POINT('Ctrl Pts',(-2.70121137800042,11.6554700696645,128.745050570368)) ;
#12165=CARTESIAN_POINT('Ctrl Pts',(-2.85184170514048,11.4748823176714,129.079612830176)) ;
#12166=CARTESIAN_POINT('Ctrl Pts',(-2.93806835347429,11.6553602398041,129.43686799927)) ;
#12167=CARTESIAN_POINT('Ctrl Pts',(-2.95399843334428,11.8778421094138,129.534266097453)) ;
#12168=CARTESIAN_POINT('Ctrl Pts',(-2.95686297599919,11.9999219050466,129.548308897304)) ;
#12169=CARTESIAN_POINT('Ctrl Pts',(-2.9541885151246,12.1224415237254,129.534619673828)) ;
#12170=CARTESIAN_POINT('Ctrl Pts',(-2.93724684308448,12.3437758281832,129.435392991623)) ;
#12171=CARTESIAN_POINT('Ctrl Pts',(-2.88852216719596,12.4517203783323,129.228824659478)) ;
#12172=CARTESIAN_POINT('Ctrl Pts',(-2.83831085827015,12.4500000000046,129.084411247894)) ;
#12173=CARTESIAN_POINT('Ctrl Pts',(2.6963321026674,12.2999451040947,130.979031266417)) ;
#12174=CARTESIAN_POINT('Ctrl Pts',(2.66563648729354,12.3010858736612,131.070864278016)) ;
#12175=CARTESIAN_POINT('Ctrl Pts',(2.60362757434741,12.229152508386,131.190957001293)) ;
#12176=CARTESIAN_POINT('Ctrl Pts',(2.56876939441479,12.0816041171335,131.24557404925)) ;
#12177=CARTESIAN_POINT('Ctrl Pts',(2.56420616301492,11.9995576103439,131.253256926599)) ;
#12178=CARTESIAN_POINT('Ctrl Pts',(2.56885622936123,11.9181473996368,131.245258218949)) ;
#12179=CARTESIAN_POINT('Ctrl Pts',(2.60376633380277,11.7701460020227,131.191527526079)) ;
#12180=CARTESIAN_POINT('Ctrl Pts',(2.70920033301593,11.6499866682161,130.983540223053)) ;
#12181=CARTESIAN_POINT('Ctrl Pts',(2.75357841904063,11.7702819290618,130.753829963316)) ;
#12182=CARTESIAN_POINT('Ctrl Pts',(2.758728952533,11.9185765432388,130.690466270959)) ;
#12183=CARTESIAN_POINT('Ctrl Pts',(2.75999631694092,12.0003485349743,130.681342359721)) ;
#12184=CARTESIAN_POINT('Ctrl Pts',(2.75885870872237,12.0820111503522,130.690378302155)) ;
#12185=CARTESIAN_POINT('Ctrl Pts',(2.75289914346115,12.2293524229409,130.755122466735)) ;
#12186=CARTESIAN_POINT('Ctrl Pts',(2.72834618207466,12.3010911231439,130.887661418871)) ;
#12187=CARTESIAN_POINT('Ctrl Pts',(2.6963321026674,12.2999451040947,130.979031266417)) ;
#12188=CARTESIAN_POINT('Ctrl Pts',(2.83829898912097,12.45,131.027630391263)) ;
#12189=CARTESIAN_POINT('Ctrl Pts',(2.78947280025513,12.4517114687695,131.172541087384)) ;
#12190=CARTESIAN_POINT('Ctrl Pts',(2.70139471334048,12.3437916712311,131.365573723284)) ;
#12191=CARTESIAN_POINT('Ctrl Pts',(2.65396227551661,12.1224285785616,131.454437395721)) ;
#12192=CARTESIAN_POINT('Ctrl Pts',(2.64766695170644,11.999336294049,131.466882783976)) ;
#12193=CARTESIAN_POINT('Ctrl Pts',(2.65410944362262,11.8771986284416,131.453942044738)) ;
#12194=CARTESIAN_POINT('Ctrl Pts',(2.70145638019102,11.6551559015813,131.366420835457)) ;
#12195=CARTESIAN_POINT('Ctrl Pts',(2.85182798968834,11.4748839115138,131.032425729989)) ;
#12196=CARTESIAN_POINT('Ctrl Pts',(2.93806166665439,11.6553598295364,130.675176301307)) ;
#12197=CARTESIAN_POINT('Ctrl Pts',(2.95399268904346,11.8778424616273,130.577776192786)) ;
#12198=CARTESIAN_POINT('Ctrl Pts',(2.95686908638074,12.0005228981401,130.563666450679)) ;
#12199=CARTESIAN_POINT('Ctrl Pts',(2.95415063990756,12.123039240118,130.577621186444)) ;
#12200=CARTESIAN_POINT('Ctrl Pts',(2.93710053667241,12.3440915979847,130.677255743497)) ;
#12201=CARTESIAN_POINT('Ctrl Pts',(2.88851115280989,12.4517193443413,130.883212820616)) ;
#12202=CARTESIAN_POINT('Ctrl Pts',(2.83829898912097,12.45,131.027630391263)) ;
#12203=CARTESIAN_POINT('',(2.83829898912097,12.45,131.027630391263)) ;
#12204=CARTESIAN_POINT('',(2.69638403966492,12.3,130.979049045863)) ;
#12205=CARTESIAN_POINT('Ctrl Pts',(2.83829898912097,12.45,131.027630391263)) ;
#12206=CARTESIAN_POINT('Ctrl Pts',(2.78947280025513,12.4517114687695,131.172541087384)) ;
#12207=CARTESIAN_POINT('Ctrl Pts',(2.70139471334048,12.3437916712311,131.365573723284)) ;
#12208=CARTESIAN_POINT('Ctrl Pts',(2.65396227551661,12.1224285785616,131.454437395721)) ;
#12209=CARTESIAN_POINT('Ctrl Pts',(2.64766695170644,11.999336294049,131.466882783976)) ;
#12210=CARTESIAN_POINT('Ctrl Pts',(2.65410944362262,11.8771986284416,131.453942044738)) ;
#12211=CARTESIAN_POINT('Ctrl Pts',(2.70145638019102,11.6551559015813,131.366420835457)) ;
#12212=CARTESIAN_POINT('Ctrl Pts',(2.85182798968834,11.4748839115138,131.032425729989)) ;
#12213=CARTESIAN_POINT('Ctrl Pts',(2.93806166665439,11.6553598295364,130.675176301307)) ;
#12214=CARTESIAN_POINT('Ctrl Pts',(2.95399268904346,11.8778424616273,130.577776192786)) ;
#12215=CARTESIAN_POINT('Ctrl Pts',(2.95686908638074,12.0005228981401,130.563666450679)) ;
#12216=CARTESIAN_POINT('Ctrl Pts',(2.95415063990756,12.123039240118,130.577621186444)) ;
#12217=CARTESIAN_POINT('Ctrl Pts',(2.93710053667241,12.3440915979847,130.677255743497)) ;
#12218=CARTESIAN_POINT('Ctrl Pts',(2.88851115280989,12.4517193443413,130.883212820616)) ;
#12219=CARTESIAN_POINT('Ctrl Pts',(2.83829898912097,12.45,131.027630391263)) ;
#12220=CARTESIAN_POINT('Ctrl Pts',(-2.69634337775187,-12.2999451036814,
129.133008638608)) ;
#12221=CARTESIAN_POINT('Ctrl Pts',(-2.72836499658603,-12.3010858731961,
129.224387732003)) ;
#12222=CARTESIAN_POINT('Ctrl Pts',(-2.75296065854718,-12.2291525080769,
129.357287772783)) ;
#12223=CARTESIAN_POINT('Ctrl Pts',(-2.75888597978306,-12.0816041170245,
129.421809127302)) ;
#12224=CARTESIAN_POINT('Ctrl Pts',(-2.75998831777564,-11.9995576103479,
129.430676738931)) ;
#12225=CARTESIAN_POINT('Ctrl Pts',(-2.75876104868106,-11.9181473997497,
129.421506338094)) ;
#12226=CARTESIAN_POINT('Ctrl Pts',(-2.75341994188481,-11.7701460023394,
129.357653575336)) ;
#12227=CARTESIAN_POINT('Ctrl Pts',(-2.70927528047414,-11.6499866686978,
129.128685684283)) ;
#12228=CARTESIAN_POINT('Ctrl Pts',(-2.60357079350359,-11.7702819293804,
128.91996870082)) ;
#12229=CARTESIAN_POINT('Ctrl Pts',(-2.56880981077416,-11.9185765433525,
128.866741268284)) ;
#12230=CARTESIAN_POINT('Ctrl Pts',(-2.5642199185338,-12.000348534976,128.858754726001)) ;
#12231=CARTESIAN_POINT('Ctrl Pts',(-2.5688584365676,-12.082011150236,128.866592235696)) ;
#12232=CARTESIAN_POINT('Ctrl Pts',(-2.60382610039754,-12.2293524226308,
128.921406337355)) ;
#12233=CARTESIAN_POINT('Ctrl Pts',(-2.66564747078675,-12.3010911227233,
129.041187553936)) ;
#12234=CARTESIAN_POINT('Ctrl Pts',(-2.69634337775187,-12.2999451036814,
129.133008638608)) ;
#12235=CARTESIAN_POINT('Ctrl Pts',(-2.83831085827053,-12.4500000000046,
129.084411247895)) ;
#12236=CARTESIAN_POINT('Ctrl Pts',(-2.88853286687405,-12.4517114685942,
129.22884412645)) ;
#12237=CARTESIAN_POINT('Ctrl Pts',(-2.93722782612733,-12.3437916712762,
129.435358408931)) ;
#12238=CARTESIAN_POINT('Ctrl Pts',(-2.95420403662341,-12.122428578556,129.534647868183)) ;
#12239=CARTESIAN_POINT('Ctrl Pts',(-2.95685624455285,-11.9993362940612,
129.548340369185)) ;
#12240=CARTESIAN_POINT('Ctrl Pts',(-2.9540167665531,-11.877198628427,129.534166244923)) ;
#12241=CARTESIAN_POINT('Ctrl Pts',(-2.93779569001346,-11.6551559016217,
129.435990019905)) ;
#12242=CARTESIAN_POINT('Ctrl Pts',(-2.85194041548293,-11.4748839115136,
129.079909659282)) ;
#12243=CARTESIAN_POINT('Ctrl Pts',(-2.70115138870184,-11.6553598294949,
128.744758841329)) ;
#12244=CARTESIAN_POINT('Ctrl Pts',(-2.65405087213571,-11.8778424616459,
128.658028685406)) ;
#12245=CARTESIAN_POINT('Ctrl Pts',(-2.64767700965671,-12.000522898136,128.645116196827)) ;
#12246=CARTESIAN_POINT('Ctrl Pts',(-2.65408069536962,-12.1230392401235,
128.657809400166)) ;
#12247=CARTESIAN_POINT('Ctrl Pts',(-2.70166622738757,-12.3440915979617,
128.746991058121)) ;
#12248=CARTESIAN_POINT('Ctrl Pts',(-2.78948627088357,-12.4517193444251,
128.939518681633)) ;
#12249=CARTESIAN_POINT('Ctrl Pts',(-2.83831085827053,-12.4500000000046,
129.084411247895)) ;
#12250=CARTESIAN_POINT('',(-2.83831085827053,-12.4500000000046,129.084411247895)) ;
#12251=CARTESIAN_POINT('',(-2.69639531535755,-12.3,129.132990859662)) ;
#12252=CARTESIAN_POINT('Ctrl Pts',(-2.83831085827053,-12.4500000000046,
129.084411247895)) ;
#12253=CARTESIAN_POINT('Ctrl Pts',(-2.88853286687405,-12.4517114685942,
129.22884412645)) ;
#12254=CARTESIAN_POINT('Ctrl Pts',(-2.93722782612733,-12.3437916712762,
129.435358408931)) ;
#12255=CARTESIAN_POINT('Ctrl Pts',(-2.95420403662341,-12.122428578556,129.534647868183)) ;
#12256=CARTESIAN_POINT('Ctrl Pts',(-2.95685624455285,-11.9993362940612,
129.548340369185)) ;
#12257=CARTESIAN_POINT('Ctrl Pts',(-2.9540167665531,-11.877198628427,129.534166244923)) ;
#12258=CARTESIAN_POINT('Ctrl Pts',(-2.93779569001346,-11.6551559016217,
129.435990019905)) ;
#12259=CARTESIAN_POINT('Ctrl Pts',(-2.85194041548293,-11.4748839115136,
129.079909659282)) ;
#12260=CARTESIAN_POINT('Ctrl Pts',(-2.70115138870184,-11.6553598294949,
128.744758841329)) ;
#12261=CARTESIAN_POINT('Ctrl Pts',(-2.65405087213571,-11.8778424616459,
128.658028685406)) ;
#12262=CARTESIAN_POINT('Ctrl Pts',(-2.64767700965671,-12.000522898136,128.645116196827)) ;
#12263=CARTESIAN_POINT('Ctrl Pts',(-2.65408069536962,-12.1230392401235,
128.657809400166)) ;
#12264=CARTESIAN_POINT('Ctrl Pts',(-2.70166622738757,-12.3440915979617,
128.746991058121)) ;
#12265=CARTESIAN_POINT('Ctrl Pts',(-2.78948627088357,-12.4517193444251,
128.939518681633)) ;
#12266=CARTESIAN_POINT('Ctrl Pts',(-2.83831085827053,-12.4500000000046,
129.084411247895)) ;
#12267=CARTESIAN_POINT('Ctrl Pts',(2.69633205354012,-12.2999450521686,130.979031249599)) ;
#12268=CARTESIAN_POINT('Ctrl Pts',(2.72835348567343,-12.3010848681391,130.887649149123)) ;
#12269=CARTESIAN_POINT('Ctrl Pts',(2.75288606391975,-12.2293633531313,130.755144199488)) ;
#12270=CARTESIAN_POINT('Ctrl Pts',(2.75886920933641,-12.082002231396,130.690360713879)) ;
#12271=CARTESIAN_POINT('Ctrl Pts',(2.75998307604284,-12.000359613974,130.681364400907)) ;
#12272=CARTESIAN_POINT('Ctrl Pts',(2.75876427003582,-11.918547034261,130.690406873977)) ;
#12273=CARTESIAN_POINT('Ctrl Pts',(2.75348410569851,-11.7703549557434,130.753996321671)) ;
#12274=CARTESIAN_POINT('Ctrl Pts',(2.70926597240985,-11.64998584046,130.983353308347)) ;
#12275=CARTESIAN_POINT('Ctrl Pts',(2.60373618782364,-11.7700747434147,131.191714976771)) ;
#12276=CARTESIAN_POINT('Ctrl Pts',(2.56886561000273,-11.9181762331761,131.245190263093)) ;
#12277=CARTESIAN_POINT('Ctrl Pts',(2.56420273427314,-11.9995468614726,131.253281856879)) ;
#12278=CARTESIAN_POINT('Ctrl Pts',(2.5687721064189,-12.0816128339373,131.245553724604)) ;
#12279=CARTESIAN_POINT('Ctrl Pts',(2.60362416609314,-12.2291417112777,131.190981884302)) ;
#12280=CARTESIAN_POINT('Ctrl Pts',(2.66563834676689,-12.3010918886182,131.070850177172)) ;
#12281=CARTESIAN_POINT('Ctrl Pts',(2.69633205354012,-12.2999450521686,130.979031249599)) ;
#12282=CARTESIAN_POINT('Ctrl Pts',(2.83829898912097,-12.45,131.027630391263)) ;
#12283=CARTESIAN_POINT('Ctrl Pts',(2.88852128598129,-12.4517100383197,130.883192931152)) ;
#12284=CARTESIAN_POINT('Ctrl Pts',(2.93708261399409,-12.3441080558366,130.677290924386)) ;
#12285=CARTESIAN_POINT('Ctrl Pts',(2.95416519277115,-12.1230258805381,130.577592616342)) ;
#12286=CARTESIAN_POINT('Ctrl Pts',(2.95685094224693,-12.0005395197688,130.56370210597)) ;
#12287=CARTESIAN_POINT('Ctrl Pts',(2.95404148282776,-11.8777981689198,130.577679899858)) ;
#12288=CARTESIAN_POINT('Ctrl Pts',(2.93793040819287,-11.6554693299226,130.675445005759)) ;
#12289=CARTESIAN_POINT('Ctrl Pts',(2.85193092472614,-11.4748825787485,131.032130289841)) ;
#12290=CARTESIAN_POINT('Ctrl Pts',(2.70139276112938,-11.6550489344215,131.366711469615)) ;
#12291=CARTESIAN_POINT('Ctrl Pts',(2.65413082319135,-11.8772418654012,131.453837068699)) ;
#12292=CARTESIAN_POINT('Ctrl Pts',(2.64765915018694,-11.9993201676784,131.466921440071)) ;
#12293=CARTESIAN_POINT('Ctrl Pts',(2.65396858084,-12.1224416773533,131.454406087865)) ;
#12294=CARTESIAN_POINT('Ctrl Pts',(2.70138694980991,-12.3437755321235,131.365612282658)) ;
#12295=CARTESIAN_POINT('Ctrl Pts',(2.78947717755393,-12.4517205710547,131.17251934375)) ;
#12296=CARTESIAN_POINT('Ctrl Pts',(2.83829898912097,-12.45,131.027630391263)) ;
#12297=CARTESIAN_POINT('',(2.83829898912098,-12.45,131.027630391263)) ;
#12298=CARTESIAN_POINT('',(2.69638403966492,-12.3,130.979049045863)) ;
#12299=CARTESIAN_POINT('Ctrl Pts',(2.83829898912097,-12.45,131.027630391263)) ;
#12300=CARTESIAN_POINT('Ctrl Pts',(2.88852128598129,-12.4517100383197,130.883192931152)) ;
#12301=CARTESIAN_POINT('Ctrl Pts',(2.93708261399409,-12.3441080558366,130.677290924386)) ;
#12302=CARTESIAN_POINT('Ctrl Pts',(2.95416519277115,-12.1230258805381,130.577592616342)) ;
#12303=CARTESIAN_POINT('Ctrl Pts',(2.95685094224693,-12.0005395197688,130.56370210597)) ;
#12304=CARTESIAN_POINT('Ctrl Pts',(2.95404148282776,-11.8777981689198,130.577679899858)) ;
#12305=CARTESIAN_POINT('Ctrl Pts',(2.93793040819287,-11.6554693299226,130.675445005759)) ;
#12306=CARTESIAN_POINT('Ctrl Pts',(2.85193092472614,-11.4748825787485,131.032130289841)) ;
#12307=CARTESIAN_POINT('Ctrl Pts',(2.70139276112938,-11.6550489344215,131.366711469615)) ;
#12308=CARTESIAN_POINT('Ctrl Pts',(2.65413082319135,-11.8772418654012,131.453837068699)) ;
#12309=CARTESIAN_POINT('Ctrl Pts',(2.64765915018694,-11.9993201676784,131.466921440071)) ;
#12310=CARTESIAN_POINT('Ctrl Pts',(2.65396858084,-12.1224416773533,131.454406087865)) ;
#12311=CARTESIAN_POINT('Ctrl Pts',(2.70138694980991,-12.3437755321235,131.365612282658)) ;
#12312=CARTESIAN_POINT('Ctrl Pts',(2.78947717755393,-12.4517205710547,131.17251934375)) ;
#12313=CARTESIAN_POINT('Ctrl Pts',(2.83829898912097,-12.45,131.027630391263)) ;
#12314=CARTESIAN_POINT('Origin',(5.27355936696949E-15,100.00000000005,130.056003483261)) ;
#12315=CARTESIAN_POINT('',(0.643026455659758,99.8500000000496,132.986279404965)) ;
#12316=CARTESIAN_POINT('Origin',(-1.36002320516582E-14,99.8500000000496,
130.056003483261)) ;
#12317=CARTESIAN_POINT('',(0.643026455659758,-99.8499999999504,132.986279404965)) ;
#12318=CARTESIAN_POINT('',(0.643026455659782,100.00000000005,132.986279404965)) ;
#12319=CARTESIAN_POINT('Origin',(-1.12410081243297E-14,-99.8499999999504,
130.056003483261)) ;
#12320=CARTESIAN_POINT('Origin',(0.643026455659758,100.00000000005,132.986279404965)) ;
#12321=CARTESIAN_POINT('',(0.610875132876776,100.00000000005,132.83976560888)) ;
#12322=CARTESIAN_POINT('Ctrl Pts',(0.610875132876776,100.00000000005,132.83976560888)) ;
#12323=CARTESIAN_POINT('Ctrl Pts',(0.246570545573965,100.00000000005,132.91992659085)) ;
#12324=CARTESIAN_POINT('Ctrl Pts',(-0.513976097476131,100.00000000005,132.934697342956)) ;
#12325=CARTESIAN_POINT('Ctrl Pts',(-1.57650948054571,100.00000000005,132.518992741361)) ;
#12326=CARTESIAN_POINT('Ctrl Pts',(-2.39903957015677,100.00000000005,131.728143423236)) ;
#12327=CARTESIAN_POINT('Ctrl Pts',(-2.85632478451787,100.00000000005,130.68282018298)) ;
#12328=CARTESIAN_POINT('Ctrl Pts',(-2.87877507902931,100.00000000005,129.542025478823)) ;
#12329=CARTESIAN_POINT('Ctrl Pts',(-2.46294820116718,100.00000000005,128.479497242434)) ;
#12330=CARTESIAN_POINT('Ctrl Pts',(-1.67216208711123,100.000000000049,127.656961864287)) ;
#12331=CARTESIAN_POINT('Ctrl Pts',(-0.626804505408765,100.00000000005,127.199679863034)) ;
#12332=CARTESIAN_POINT('Ctrl Pts',(0.513970981949363,100.000000000049,127.177227729026)) ;
#12333=CARTESIAN_POINT('Ctrl Pts',(1.57651021040797,100.00000000005,127.593055664409)) ;
#12334=CARTESIAN_POINT('Ctrl Pts',(2.39903942226395,100.00000000005,128.383841184256)) ;
#12335=CARTESIAN_POINT('Ctrl Pts',(2.85632483652517,100.00000000005,129.429199095725)) ;
#12336=CARTESIAN_POINT('Ctrl Pts',(2.8787739006122,100.00000000005,130.569976264547)) ;
#12337=CARTESIAN_POINT('Ctrl Pts',(2.462957930535,100.00000000005,131.632548023818)) ;
#12338=CARTESIAN_POINT('Ctrl Pts',(1.67212837843037,100.000000000049,132.454981361557)) ;
#12339=CARTESIAN_POINT('Ctrl Pts',(0.975293053555267,100.00000000005,132.760016407974)) ;
#12340=CARTESIAN_POINT('Ctrl Pts',(0.610875132876776,100.00000000005,132.83976560888)) ;
#12341=CARTESIAN_POINT('Origin',(0.643026455659758,-99.9999999999504,132.986279404965)) ;
#12342=CARTESIAN_POINT('',(0.610875132876776,-99.9999999999504,132.83976560888)) ;
#12343=CARTESIAN_POINT('Ctrl Pts',(0.610875132876776,-99.9999999999504,
132.83976560888)) ;
#12344=CARTESIAN_POINT('Ctrl Pts',(0.246570545573981,-99.9999999999506,
132.919926590851)) ;
#12345=CARTESIAN_POINT('Ctrl Pts',(-0.513976097476131,-99.9999999999504,
132.934697342956)) ;
#12346=CARTESIAN_POINT('Ctrl Pts',(-1.57650948054572,-99.9999999999505,
132.518992741361)) ;
#12347=CARTESIAN_POINT('Ctrl Pts',(-2.39903957015677,-99.9999999999504,
131.728143423236)) ;
#12348=CARTESIAN_POINT('Ctrl Pts',(-2.85632478451788,-99.9999999999505,
130.68282018298)) ;
#12349=CARTESIAN_POINT('Ctrl Pts',(-2.87877507896514,-99.9999999999504,
129.542025478827)) ;
#12350=CARTESIAN_POINT('Ctrl Pts',(-2.46294820107204,-99.9999999999504,
128.479497242403)) ;
#12351=CARTESIAN_POINT('Ctrl Pts',(-1.67216208741986,-99.9999999999505,
127.656961864367)) ;
#12352=CARTESIAN_POINT('Ctrl Pts',(-0.626804504682387,-99.9999999999505,
127.199679862876)) ;
#12353=CARTESIAN_POINT('Ctrl Pts',(0.513970981616631,-99.9999999999502,
127.177227729086)) ;
#12354=CARTESIAN_POINT('Ctrl Pts',(1.5765102105793,-99.9999999999503,127.593055664377)) ;
#12355=CARTESIAN_POINT('Ctrl Pts',(2.39903942217006,-99.9999999999505,128.383841184273)) ;
#12356=CARTESIAN_POINT('Ctrl Pts',(2.85632483657695,-99.9999999999504,129.429199095716)) ;
#12357=CARTESIAN_POINT('Ctrl Pts',(2.87877390058261,-99.9999999999505,130.569976264552)) ;
#12358=CARTESIAN_POINT('Ctrl Pts',(2.46295793055283,-99.9999999999503,131.632548023814)) ;
#12359=CARTESIAN_POINT('Ctrl Pts',(1.67212837841725,-99.9999999999505,132.45498136156)) ;
#12360=CARTESIAN_POINT('Ctrl Pts',(0.975293053561667,-99.9999999999504,
132.760016407972)) ;
#12361=CARTESIAN_POINT('Ctrl Pts',(0.610875132876776,-99.9999999999504,
132.83976560888)) ;
#12362=CARTESIAN_POINT('Ctrl Pts',(0.643026455659758,99.8500000000496,132.986279404965)) ;
#12363=CARTESIAN_POINT('Ctrl Pts',(0.259547942953796,99.8500000000496,133.070659386104)) ;
#12364=CARTESIAN_POINT('Ctrl Pts',(-0.541027471492163,99.8500000000496,
133.086207545669)) ;
#12365=CARTESIAN_POINT('Ctrl Pts',(-1.65948366334539,99.8500000000496,132.648623755083)) ;
#12366=CARTESIAN_POINT('Ctrl Pts',(-2.52530481091486,99.8500000000496,131.816150788913)) ;
#12367=CARTESIAN_POINT('Ctrl Pts',(-3.00665766787806,99.8500000000497,130.715810534794)) ;
#12368=CARTESIAN_POINT('Ctrl Pts',(-3.03028955669294,99.8500000000495,129.514974005128)) ;
#12369=CARTESIAN_POINT('Ctrl Pts',(-2.59257705385615,99.8500000000497,128.396523229773)) ;
#12370=CARTESIAN_POINT('Ctrl Pts',(-1.76017061831144,99.8500000000494,127.530696516006)) ;
#12371=CARTESIAN_POINT('Ctrl Pts',(-0.659794215338994,99.8500000000498,
127.049347040875)) ;
#12372=CARTESIAN_POINT('Ctrl Pts',(0.541022085740472,99.8500000000495,127.025713215585)) ;
#12373=CARTESIAN_POINT('Ctrl Pts',(1.6594844324448,99.8500000000496,127.463426831923)) ;
#12374=CARTESIAN_POINT('Ctrl Pts',(2.52530465476544,99.8500000000496,128.295832642362)) ;
#12375=CARTESIAN_POINT('Ctrl Pts',(3.00665772253955,99.8500000000496,129.396209390568)) ;
#12376=CARTESIAN_POINT('Ctrl Pts',(3.03028831652775,99.8500000000497,130.597027463672)) ;
#12377=CARTESIAN_POINT('Ctrl Pts',(2.59258729503993,99.8500000000496,131.715524052452)) ;
#12378=CARTESIAN_POINT('Ctrl Pts',(1.76013513546983,99.8500000000496,132.581243354859)) ;
#12379=CARTESIAN_POINT('Ctrl Pts',(1.02662426675004,99.8500000000496,132.902332877864)) ;
#12380=CARTESIAN_POINT('Ctrl Pts',(0.643026455659758,99.8500000000496,132.986279404965)) ;
#12381=CARTESIAN_POINT('Ctrl Pts',(0.610875132876776,100.00000000005,132.83976560888)) ;
#12382=CARTESIAN_POINT('Ctrl Pts',(0.246570545573965,100.00000000005,132.91992659085)) ;
#12383=CARTESIAN_POINT('Ctrl Pts',(-0.513976097476131,100.00000000005,132.934697342956)) ;
#12384=CARTESIAN_POINT('Ctrl Pts',(-1.57650948054571,100.00000000005,132.518992741361)) ;
#12385=CARTESIAN_POINT('Ctrl Pts',(-2.39903957015677,100.00000000005,131.728143423236)) ;
#12386=CARTESIAN_POINT('Ctrl Pts',(-2.85632478451787,100.00000000005,130.68282018298)) ;
#12387=CARTESIAN_POINT('Ctrl Pts',(-2.87877507902931,100.00000000005,129.542025478823)) ;
#12388=CARTESIAN_POINT('Ctrl Pts',(-2.46294820116718,100.00000000005,128.479497242434)) ;
#12389=CARTESIAN_POINT('Ctrl Pts',(-1.67216208711123,100.000000000049,127.656961864287)) ;
#12390=CARTESIAN_POINT('Ctrl Pts',(-0.626804505408765,100.00000000005,127.199679863034)) ;
#12391=CARTESIAN_POINT('Ctrl Pts',(0.513970981949363,100.000000000049,127.177227729026)) ;
#12392=CARTESIAN_POINT('Ctrl Pts',(1.57651021040797,100.00000000005,127.593055664409)) ;
#12393=CARTESIAN_POINT('Ctrl Pts',(2.39903942226395,100.00000000005,128.383841184256)) ;
#12394=CARTESIAN_POINT('Ctrl Pts',(2.85632483652517,100.00000000005,129.429199095725)) ;
#12395=CARTESIAN_POINT('Ctrl Pts',(2.8787739006122,100.00000000005,130.569976264547)) ;
#12396=CARTESIAN_POINT('Ctrl Pts',(2.462957930535,100.00000000005,131.632548023818)) ;
#12397=CARTESIAN_POINT('Ctrl Pts',(1.67212837843037,100.000000000049,132.454981361557)) ;
#12398=CARTESIAN_POINT('Ctrl Pts',(0.975293053555267,100.00000000005,132.760016407974)) ;
#12399=CARTESIAN_POINT('Ctrl Pts',(0.610875132876776,100.00000000005,132.83976560888)) ;
#12400=CARTESIAN_POINT('',(0.643026455659758,99.8500000000496,132.986279404965)) ;
#12401=CARTESIAN_POINT('Ctrl Pts',(0.643026455659758,-99.8499999999504,
132.986279404965)) ;
#12402=CARTESIAN_POINT('Ctrl Pts',(0.610875132876776,-99.9999999999504,
132.83976560888)) ;
#12403=CARTESIAN_POINT('Ctrl Pts',(0.259547942953806,-99.8499999999506,
133.070659386104)) ;
#12404=CARTESIAN_POINT('Ctrl Pts',(0.246570545573981,-99.9999999999506,
132.919926590851)) ;
#12405=CARTESIAN_POINT('Ctrl Pts',(-0.541027471492161,-99.8499999999503,
133.086207545669)) ;
#12406=CARTESIAN_POINT('Ctrl Pts',(-0.513976097476131,-99.9999999999504,
132.934697342956)) ;
#12407=CARTESIAN_POINT('Ctrl Pts',(-1.6594836633454,-99.8499999999505,132.648623755083)) ;
#12408=CARTESIAN_POINT('Ctrl Pts',(-1.57650948054572,-99.9999999999505,
132.518992741361)) ;
#12409=CARTESIAN_POINT('Ctrl Pts',(-2.52530481091486,-99.8499999999504,
131.816150788913)) ;
#12410=CARTESIAN_POINT('Ctrl Pts',(-2.39903957015677,-99.9999999999504,
131.728143423236)) ;
#12411=CARTESIAN_POINT('Ctrl Pts',(-3.00665766787808,-99.8499999999505,
130.715810534794)) ;
#12412=CARTESIAN_POINT('Ctrl Pts',(-2.85632478451788,-99.9999999999505,
130.68282018298)) ;
#12413=CARTESIAN_POINT('Ctrl Pts',(-3.03028955675574,-99.8499999999505,
129.514974005143)) ;
#12414=CARTESIAN_POINT('Ctrl Pts',(-2.87877507896514,-99.9999999999504,
129.542025478827)) ;
#12415=CARTESIAN_POINT('Ctrl Pts',(-2.59257705395858,-99.8499999999503,
128.396523229796)) ;
#12416=CARTESIAN_POINT('Ctrl Pts',(-2.46294820107204,-99.9999999999504,
128.479497242403)) ;
#12417=CARTESIAN_POINT('Ctrl Pts',(-1.76017061799586,-99.8499999999505,
127.53069651594)) ;
#12418=CARTESIAN_POINT('Ctrl Pts',(-1.67216208741986,-99.9999999999505,
127.656961864367)) ;
#12419=CARTESIAN_POINT('Ctrl Pts',(-0.659794216106477,-99.8499999999505,
127.049347041044)) ;
#12420=CARTESIAN_POINT('Ctrl Pts',(-0.626804504682387,-99.9999999999505,
127.199679862876)) ;
#12421=CARTESIAN_POINT('Ctrl Pts',(0.541022086074333,-99.8499999999503,
127.025713215508)) ;
#12422=CARTESIAN_POINT('Ctrl Pts',(0.513970981616631,-99.9999999999502,
127.177227729086)) ;
#12423=CARTESIAN_POINT('Ctrl Pts',(1.65948443226611,-99.8499999999503,127.463426831961)) ;
#12424=CARTESIAN_POINT('Ctrl Pts',(1.5765102105793,-99.9999999999503,127.593055664377)) ;
#12425=CARTESIAN_POINT('Ctrl Pts',(2.52530465486198,-99.8499999999505,128.295832642341)) ;
#12426=CARTESIAN_POINT('Ctrl Pts',(2.39903942217006,-99.9999999999505,128.383841184273)) ;
#12427=CARTESIAN_POINT('Ctrl Pts',(3.00665772248627,-99.8499999999503,129.39620939058)) ;
#12428=CARTESIAN_POINT('Ctrl Pts',(2.85632483657695,-99.9999999999504,129.429199095716)) ;
#12429=CARTESIAN_POINT('Ctrl Pts',(3.03028831655821,-99.8499999999504,130.597027463665)) ;
#12430=CARTESIAN_POINT('Ctrl Pts',(2.87877390058261,-99.9999999999505,130.569976264552)) ;
#12431=CARTESIAN_POINT('Ctrl Pts',(2.59258729502161,-99.8499999999503,131.715524052456)) ;
#12432=CARTESIAN_POINT('Ctrl Pts',(2.46295793055283,-99.9999999999503,131.632548023814)) ;
#12433=CARTESIAN_POINT('Ctrl Pts',(1.76013513548333,-99.8499999999505,132.581243354857)) ;
#12434=CARTESIAN_POINT('Ctrl Pts',(1.67212837841725,-99.9999999999505,132.45498136156)) ;
#12435=CARTESIAN_POINT('Ctrl Pts',(1.02662426674344,-99.8499999999505,132.902332877865)) ;
#12436=CARTESIAN_POINT('Ctrl Pts',(0.975293053561667,-99.9999999999504,
132.760016407972)) ;
#12437=CARTESIAN_POINT('Ctrl Pts',(0.643026455659758,-99.8499999999504,
132.986279404965)) ;
#12438=CARTESIAN_POINT('Ctrl Pts',(0.610875132876776,-99.9999999999504,
132.83976560888)) ;
#12439=CARTESIAN_POINT('',(0.643026455659758,-99.8499999999504,132.986279404965)) ;
#196737=UNCERTAINTY_MEASURE_WITH_UNIT(LENGTH_MEASURE(0.01),#196742,
'DISTANCE_ACCURACY_VALUE',
'Maximum model space distance between geometric entities at asserted c
onnectivities') ;
#196738=UNCERTAINTY_MEASURE_WITH_UNIT(LENGTH_MEASURE(0.01),#196742,
'DISTANCE_ACCURACY_VALUE',
'Maximum model space distance between geometric entities at asserted c
onnectivities') ;
#196740=(
GEOMETRIC_REPRESENTATION_CONTEXT(3)
GLOBAL_UNCERTAINTY_ASSIGNED_CONTEXT((#196737))
GLOBAL_UNIT_ASSIGNED_CONTEXT((#196742,#196744,#196745))
REPRESENTATION_CONTEXT('','3D')
) ;
#196741=(
GEOMETRIC_REPRESENTATION_CONTEXT(3)
GLOBAL_UNCERTAINTY_ASSIGNED_CONTEXT((#196738))
GLOBAL_UNIT_ASSIGNED_CONTEXT((#196742,#196744,#196745))
REPRESENTATION_CONTEXT('','3D')
) ;
#196742=(
LENGTH_UNIT()
NAMED_UNIT(*)
SI_UNIT(.MILLI.,.METRE.)
) ;
#196744=(
NAMED_UNIT(*)
PLANE_ANGLE_UNIT()
SI_UNIT($,.RADIAN.)
) ;
#196745=(
NAMED_UNIT(*)
SI_UNIT($,.STERADIAN.)
SOLID_ANGLE_UNIT()
) ;
#196753=PRODUCT_DEFINITION_CONTEXT('part definition',#196761,'design') ;
#196761=APPLICATION_CONTEXT(
'Core Data for Automotive Mechanical Design Process') ;
#196762=PRODUCT_CONTEXT('part definition',#196761,'mechanical') ;
#196765=PRESENTATION_STYLE_ASSIGNMENT((#196767)) ;
#196767=SURFACE_STYLE_USAGE(.BOTH.,#196769) ;
#196769=SURFACE_SIDE_STYLE('',(#196771)) ;
#196771=SURFACE_STYLE_FILL_AREA(#196773) ;
#196773=FILL_AREA_STYLE('Steel - Satin',(#196775)) ;
#196775=FILL_AREA_STYLE_COLOUR('Steel - Satin',#196777) ;
#196777=COLOUR_RGB('Steel - Satin', 0.09019608, 0.27058824, 0.51372549) ;
#196779=CARTESIAN_POINT ( '', ( 0.0, 0.0, 0.0 ) ) ;
#196780=DIRECTION ( '', ( 0.0, 0.0, 1.0 ) ) ;
#196781=DIRECTION ( '', ( 1.0, 0.0, 0.0 ) ) ;
#196782=AXIS2_PLACEMENT_3D ( '', #196779, #196780, #196781 ) ;
#196783=ADVANCED_BREP_SHAPE_REPRESENTATION ( 'Pendulum Rod', ( #338, #196782, #196793, #197238 ), #196740 ) ;
#196784=PRODUCT( 'Pendulum Rod', 'Pendulum Rod', '', ( #196762 ) ) ;
#196785=PRODUCT_DEFINITION_FORMATION ( '', '', #196784 ) ;
#196786=PRODUCT_DEFINITION( 'Pendulum Rod', 'Pendulum Rod', #196785, #196753 ) ;
#196787=PRODUCT_DEFINITION_SHAPE ( '', '', #196786 ) ;
#196788=SHAPE_DEFINITION_REPRESENTATION ( #196787, #196783 ) ;
#196790=CARTESIAN_POINT ( '', ( 0.0, 0.0, 0.0 ) ) ;
#196791=DIRECTION ( '', ( 0.0, 0.0, 1.0 ) ) ;
#196792=DIRECTION ( '', ( 1.0, 0.0, 0.0 ) ) ;
#196793=AXIS2_PLACEMENT_3D ( '', #196790, #196791, #196792 ) ;
#197235=CARTESIAN_POINT ( '', ( 0.0, 0.0, 0.0 ) ) ;
#197236=DIRECTION ( '', ( 0.0, 0.0, 1.0 ) ) ;
#197237=DIRECTION ( '', ( 1.0, 0.0, 0.0 ) ) ;
#197238=AXIS2_PLACEMENT_3D ( '', #197235, #197236, #197237 ) ;
ENDSEC;
END-ISO-10303-21;
